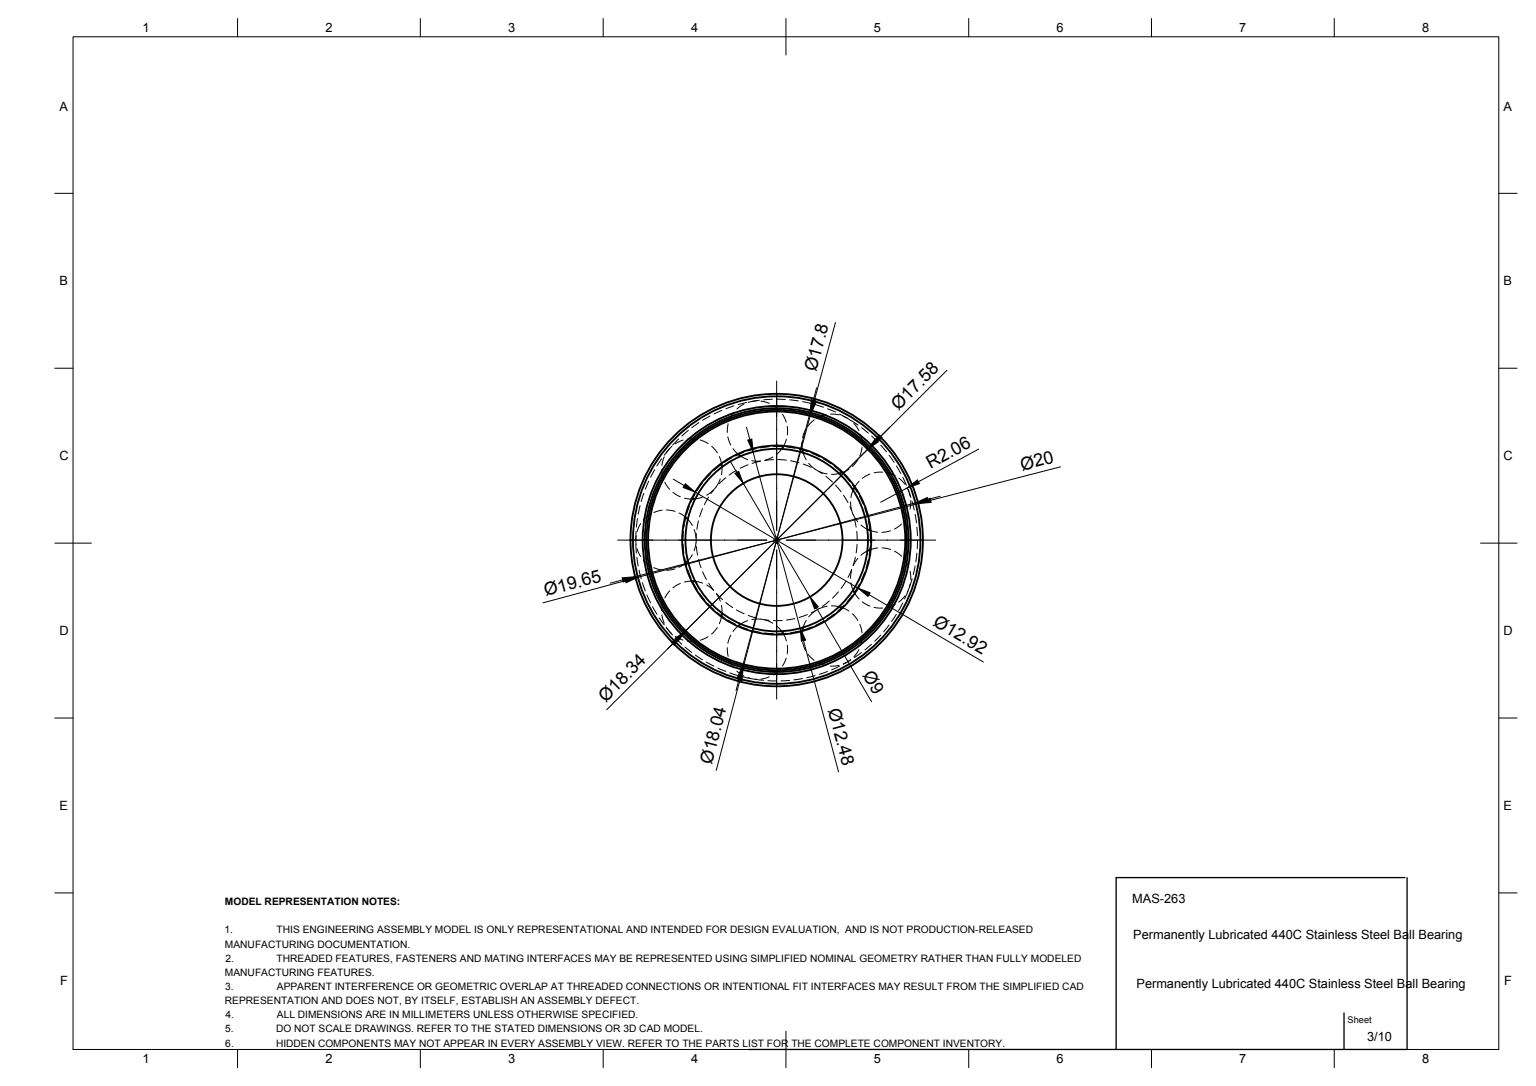
ISO-10303-21;
HEADER;
/* Generated by software containing ST-Developer
 * from STEP Tools, Inc. (www.steptools.com) 
 */

FILE_DESCRIPTION(
/* description */ (''),
/* implementation_level */ '2;1');

FILE_NAME(
/* name */ 'Permanently Lubricated 440C Stainless Steel Ball Bearing.step',
/* time_stamp */ '2026-10-12T15:47:30-07:00',
/* author */ (''),
/* organization */ (''),
/* preprocessor_version */ 'ST-DEVELOPER v20.2',
/* originating_system */ 'Autodesk Translation Framework v15.15.0.0',
/* authorisation */ '');

FILE_SCHEMA (('AUTOMOTIVE_DESIGN { 1 0 10303 214 3 1 1 }'));
ENDSEC;

DATA;
#10=MECHANICAL_DESIGN_GEOMETRIC_PRESENTATION_REPRESENTATION('',(#89,#90,#91,#92,#93,#94,#95,#96,#97,#98,#99,#100,#101,#102),#88483);
#55=SPHERICAL_SURFACE('',#14025,2.0625);
#56=SPHERICAL_SURFACE('',#14081,2.0625);
#57=SPHERICAL_SURFACE('',#14083,2.0625);
#58=SPHERICAL_SURFACE('',#14085,2.0625);
#59=SPHERICAL_SURFACE('',#14087,2.0625);
#60=SPHERICAL_SURFACE('',#14089,2.0625);
#61=SPHERICAL_SURFACE('',#14091,2.0625);
#62=SPHERICAL_SURFACE('',#14093,2.0625);
#63=SPHERICAL_SURFACE('',#14095,2.0625);
#71=SHAPE_REPRESENTATION_RELATIONSHIP('SRR','None',#88527,#80);
#80=ADVANCED_BREP_SHAPE_REPRESENTATION('',(#124,#125,#126,#127,#128,#129,
#130,#131,#132,#133,#134,#135,#136,#137),#88481);
#89=STYLED_ITEM('',(#88574),#124);
#90=STYLED_ITEM('',(#88574),#125);
#91=STYLED_ITEM('',(#88574),#126);
#92=STYLED_ITEM('',(#88574),#127);
#93=STYLED_ITEM('',(#88574),#128);
#94=STYLED_ITEM('',(#88574),#129);
#95=STYLED_ITEM('',(#88574),#130);
#96=STYLED_ITEM('',(#88574),#131);
#97=STYLED_ITEM('',(#88574),#132);
#98=STYLED_ITEM('',(#88574),#133);
#99=STYLED_ITEM('',(#88574),#134);
#100=STYLED_ITEM('',(#88574),#135);
#101=STYLED_ITEM('',(#88574),#136);
#102=STYLED_ITEM('',(#88574),#137);
#124=MANIFOLD_SOLID_BREP('Body1',#12999);
#125=MANIFOLD_SOLID_BREP('Body2',#13000);
#126=MANIFOLD_SOLID_BREP('Body3',#13001);
#127=MANIFOLD_SOLID_BREP('Body4',#13002);
#128=MANIFOLD_SOLID_BREP('Body5',#13003);
#129=MANIFOLD_SOLID_BREP('Body6',#13004);
#130=MANIFOLD_SOLID_BREP('Body7',#13005);
#131=MANIFOLD_SOLID_BREP('Body8',#13006);
#132=MANIFOLD_SOLID_BREP('Body9',#13007);
#133=MANIFOLD_SOLID_BREP('Body10',#13008);
#134=MANIFOLD_SOLID_BREP('Body11',#13009);
#135=MANIFOLD_SOLID_BREP('Body12',#13010);
#136=MANIFOLD_SOLID_BREP('Body13',#13011);
#137=MANIFOLD_SOLID_BREP('Body14',#13012);
#175=TOROIDAL_SURFACE('',#13994,7.57083333333333,2.0625);
#176=TOROIDAL_SURFACE('',#14007,5.00416666666667,0.260975870478375);
#177=TOROIDAL_SURFACE('',#14010,5.98069079618829,0.260975870478375);
#178=TOROIDAL_SURFACE('',#14017,5.98069079618829,0.260975870478375);
#179=TOROIDAL_SURFACE('',#14020,5.00416666666667,0.260975870478376);
#180=TOROIDAL_SURFACE('',#14030,6.50566666666666,0.0439999999999998);
#181=TOROIDAL_SURFACE('',#14047,6.50566666666666,0.0439999999999998);
#182=TOROIDAL_SURFACE('',#14075,7.57083333333333,2.0625);
#183=TOROIDAL_SURFACE('',#14100,6.32416666666667,0.0824999999999997);
#184=TOROIDAL_SURFACE('',#14105,6.42956528249449,0.0228986158278278);
#326=CONICAL_SURFACE('',#13998,4.5,0.26179938779915);
#327=CONICAL_SURFACE('',#14005,4.75208333333333,0.261799387799149);
#328=CONICAL_SURFACE('',#14033,8.9,0.523598775598299);
#329=CONICAL_SURFACE('',#14050,8.79,0.523598775598297);
#330=CONICAL_SURFACE('',#14054,9.01847925309041,0.349065850398861);
#331=CONICAL_SURFACE('',#14057,9.16847925309041,0.78539816339744);
#332=CONICAL_SURFACE('',#14059,10.,0.523598775598291);
#333=CONICAL_SURFACE('',#14065,9.82679491924311,0.52359877559829);
#334=CONICAL_SURFACE('',#14067,9.0184792530904,0.78539816339744);
#335=CONICAL_SURFACE('',#14070,8.9,0.349065850398861);
#336=CONICAL_SURFACE('',#14109,6.46166666666667,0.17453292519942);
#407=FACE_BOUND('',#2047,.T.);
#408=FACE_BOUND('',#2049,.T.);
#409=FACE_BOUND('',#2056,.T.);
#410=FACE_BOUND('',#2058,.T.);
#411=FACE_BOUND('',#2064,.T.);
#412=FACE_BOUND('',#2066,.T.);
#413=FACE_BOUND('',#2078,.T.);
#414=FACE_BOUND('',#2080,.T.);
#415=FACE_BOUND('',#2096,.T.);
#553=PLANE('',#14023);
#554=PLANE('',#14024);
#555=PLANE('',#14039);
#556=PLANE('',#14040);
#557=PLANE('',#14052);
#558=PLANE('',#14053);
#559=PLANE('',#14079);
#560=PLANE('',#14080);
#561=PLANE('',#14114);
#1310=FACE_OUTER_BOUND('',#2036,.T.);
#1311=FACE_OUTER_BOUND('',#2037,.T.);
#1312=FACE_OUTER_BOUND('',#2038,.T.);
#1313=FACE_OUTER_BOUND('',#2039,.T.);
#1314=FACE_OUTER_BOUND('',#2040,.T.);
#1315=FACE_OUTER_BOUND('',#2041,.T.);
#1316=FACE_OUTER_BOUND('',#2042,.T.);
#1317=FACE_OUTER_BOUND('',#2043,.T.);
#1318=FACE_OUTER_BOUND('',#2044,.T.);
#1319=FACE_OUTER_BOUND('',#2045,.T.);
#1320=FACE_OUTER_BOUND('',#2046,.T.);
#1321=FACE_OUTER_BOUND('',#2048,.T.);
#1322=FACE_OUTER_BOUND('',#2050,.T.);
#1323=FACE_OUTER_BOUND('',#2051,.T.);
#1324=FACE_OUTER_BOUND('',#2052,.T.);
#1325=FACE_OUTER_BOUND('',#2053,.T.);
#1326=FACE_OUTER_BOUND('',#2054,.T.);
#1327=FACE_OUTER_BOUND('',#2055,.T.);
#1328=FACE_OUTER_BOUND('',#2057,.T.);
#1329=FACE_OUTER_BOUND('',#2059,.T.);
#1330=FACE_OUTER_BOUND('',#2060,.T.);
#1331=FACE_OUTER_BOUND('',#2061,.T.);
#1332=FACE_OUTER_BOUND('',#2062,.T.);
#1333=FACE_OUTER_BOUND('',#2063,.T.);
#1334=FACE_OUTER_BOUND('',#2065,.T.);
#1335=FACE_OUTER_BOUND('',#2067,.T.);
#1336=FACE_OUTER_BOUND('',#2068,.T.);
#1337=FACE_OUTER_BOUND('',#2069,.T.);
#1338=FACE_OUTER_BOUND('',#2070,.T.);
#1339=FACE_OUTER_BOUND('',#2071,.T.);
#1340=FACE_OUTER_BOUND('',#2072,.T.);
#1341=FACE_OUTER_BOUND('',#2073,.T.);
#1342=FACE_OUTER_BOUND('',#2074,.T.);
#1343=FACE_OUTER_BOUND('',#2075,.T.);
#1344=FACE_OUTER_BOUND('',#2076,.T.);
#1345=FACE_OUTER_BOUND('',#2077,.T.);
#1346=FACE_OUTER_BOUND('',#2079,.T.);
#1347=FACE_OUTER_BOUND('',#2081,.T.);
#1348=FACE_OUTER_BOUND('',#2082,.T.);
#1349=FACE_OUTER_BOUND('',#2083,.T.);
#1350=FACE_OUTER_BOUND('',#2084,.T.);
#1351=FACE_OUTER_BOUND('',#2085,.T.);
#1352=FACE_OUTER_BOUND('',#2086,.T.);
#1353=FACE_OUTER_BOUND('',#2087,.T.);
#1354=FACE_OUTER_BOUND('',#2088,.T.);
#1355=FACE_OUTER_BOUND('',#2089,.T.);
#1356=FACE_OUTER_BOUND('',#2090,.T.);
#1357=FACE_OUTER_BOUND('',#2091,.T.);
#1358=FACE_OUTER_BOUND('',#2092,.T.);
#1359=FACE_OUTER_BOUND('',#2093,.T.);
#1360=FACE_OUTER_BOUND('',#2094,.T.);
#1361=FACE_OUTER_BOUND('',#2095,.T.);
#2036=EDGE_LOOP('',(#11488,#11489,#11490,#11491));
#2037=EDGE_LOOP('',(#11492,#11493,#11494,#11495,#11496,#11497));
#2038=EDGE_LOOP('',(#11498,#11499,#11500,#11501,#11502));
#2039=EDGE_LOOP('',(#11503,#11504,#11505,#11506));
#2040=EDGE_LOOP('',(#11507,#11508,#11509,#11510));
#2041=EDGE_LOOP('',(#11511,#11512,#11513,#11514));
#2042=EDGE_LOOP('',(#11515,#11516,#11517,#11518));
#2043=EDGE_LOOP('',(#11519,#11520,#11521,#11522));
#2044=EDGE_LOOP('',(#11523,#11524,#11525,#11526));
#2045=EDGE_LOOP('',(#11527,#11528,#11529,#11530,#11531));
#2046=EDGE_LOOP('',(#11532));
#2047=EDGE_LOOP('',(#11533));
#2048=EDGE_LOOP('',(#11534));
#2049=EDGE_LOOP('',(#11535));
#2050=EDGE_LOOP('',(#11536,#11537));
#2051=EDGE_LOOP('',(#11538,#11539,#11540,#11541));
#2052=EDGE_LOOP('',(#11542,#11543,#11544,#11545));
#2053=EDGE_LOOP('',(#11546,#11547,#11548,#11549,#11550));
#2054=EDGE_LOOP('',(#11551,#11552,#11553,#11554,#11555));
#2055=EDGE_LOOP('',(#11556));
#2056=EDGE_LOOP('',(#11557));
#2057=EDGE_LOOP('',(#11558));
#2058=EDGE_LOOP('',(#11559));
#2059=EDGE_LOOP('',(#11560,#11561,#11562,#11563));
#2060=EDGE_LOOP('',(#11564,#11565,#11566,#11567));
#2061=EDGE_LOOP('',(#11568,#11569,#11570,#11571));
#2062=EDGE_LOOP('',(#11572,#11573,#11574,#11575));
#2063=EDGE_LOOP('',(#11576));
#2064=EDGE_LOOP('',(#11577));
#2065=EDGE_LOOP('',(#11578));
#2066=EDGE_LOOP('',(#11579));
#2067=EDGE_LOOP('',(#11580,#11581,#11582,#11583));
#2068=EDGE_LOOP('',(#11584,#11585,#11586,#11587));
#2069=EDGE_LOOP('',(#11588,#11589,#11590,#11591,#11592));
#2070=EDGE_LOOP('',(#11593,#11594,#11595,#11596,#11597));
#2071=EDGE_LOOP('',(#11598,#11599,#11600,#11601));
#2072=EDGE_LOOP('',(#11602,#11603,#11604,#11605));
#2073=EDGE_LOOP('',(#11606,#11607,#11608,#11609,#11610));
#2074=EDGE_LOOP('',(#11611,#11612,#11613,#11614,#11615));
#2075=EDGE_LOOP('',(#11616,#11617,#11618,#11619));
#2076=EDGE_LOOP('',(#11620,#11621,#11622,#11623));
#2077=EDGE_LOOP('',(#11624));
#2078=EDGE_LOOP('',(#11625));
#2079=EDGE_LOOP('',(#11626));
#2080=EDGE_LOOP('',(#11627));
#2081=EDGE_LOOP('',(#11628,#11629));
#2082=EDGE_LOOP('',(#11630,#11631));
#2083=EDGE_LOOP('',(#11632,#11633));
#2084=EDGE_LOOP('',(#11634,#11635));
#2085=EDGE_LOOP('',(#11636,#11637));
#2086=EDGE_LOOP('',(#11638,#11639));
#2087=EDGE_LOOP('',(#11640,#11641));
#2088=EDGE_LOOP('',(#11642,#11643));
#2089=EDGE_LOOP('',(#11644,#11645,#11646,#11647));
#2090=EDGE_LOOP('',(#11648,#11649,#11650,#11651));
#2091=EDGE_LOOP('',(#11652,#11653,#11654,#11655));
#2092=EDGE_LOOP('',(#11656,#11657,#11658,#11659,#11660));
#2093=EDGE_LOOP('',(#11661,#11662,#11663,#11664,#11665,#11666));
#2094=EDGE_LOOP('',(#11667,#11668,#11669,#11670,#11671));
#2095=EDGE_LOOP('',(#11672));
#2096=EDGE_LOOP('',(#11673));
#2699=CIRCLE('',#13995,6.24166666666667);
#2700=CIRCLE('',#13996,2.0625);
#2701=CIRCLE('',#13997,6.24166666666667);
#2702=CIRCLE('',#13999,4.5);
#2703=CIRCLE('',#14000,4.75208333333333);
#2704=CIRCLE('',#14001,4.75208333333333);
#2705=CIRCLE('',#14002,4.5);
#2706=CIRCLE('',#14004,4.5);
#2707=CIRCLE('',#14006,4.75208333333333);
#2708=CIRCLE('',#14008,0.260975870478375);
#2709=CIRCLE('',#14009,5.00416666666667);
#2710=CIRCLE('',#14011,5.98069079618829);
#2711=CIRCLE('',#14012,0.260975870478375);
#2712=CIRCLE('',#14013,6.24166666666667);
#2713=CIRCLE('',#14016,6.24166666666667);
#2714=CIRCLE('',#14018,0.260975870478375);
#2715=CIRCLE('',#14019,5.98069079618829);
#2716=CIRCLE('',#14021,5.00416666666667);
#2717=CIRCLE('',#14022,0.260975870478376);
#2718=CIRCLE('',#14026,2.0625);
#2719=CIRCLE('',#14028,6.46166666666667);
#2720=CIRCLE('',#14029,6.46166666666667);
#2721=CIRCLE('',#14031,0.0439999999999998);
#2722=CIRCLE('',#14032,6.50566666666666);
#2723=CIRCLE('',#14034,8.9);
#2724=CIRCLE('',#14035,8.79);
#2725=CIRCLE('',#14036,8.9);
#2726=CIRCLE('',#14038,8.9);
#2727=CIRCLE('',#14042,8.9);
#2728=CIRCLE('',#14043,8.9);
#2729=CIRCLE('',#14045,6.46166666666667);
#2730=CIRCLE('',#14046,6.46166666666667);
#2731=CIRCLE('',#14048,6.50566666666666);
#2732=CIRCLE('',#14049,0.0439999999999998);
#2733=CIRCLE('',#14051,8.79);
#2734=CIRCLE('',#14055,8.9);
#2735=CIRCLE('',#14056,9.01847925309041);
#2736=CIRCLE('',#14058,9.16847925309041);
#2737=CIRCLE('',#14060,10.);
#2738=CIRCLE('',#14061,9.82679491924311);
#2739=CIRCLE('',#14062,10.);
#2740=CIRCLE('',#14064,10.);
#2741=CIRCLE('',#14066,9.82679491924311);
#2742=CIRCLE('',#14068,9.0184792530904);
#2743=CIRCLE('',#14069,9.1684792530904);
#2744=CIRCLE('',#14071,8.9);
#2745=CIRCLE('',#14072,8.9);
#2746=CIRCLE('',#14074,8.9);
#2747=CIRCLE('',#14076,2.0625);
#2748=CIRCLE('',#14077,8.9);
#2749=CIRCLE('',#14082,2.0625);
#2750=CIRCLE('',#14084,2.0625);
#2751=CIRCLE('',#14086,2.0625);
#2752=CIRCLE('',#14088,2.0625);
#2753=CIRCLE('',#14090,2.0625);
#2754=CIRCLE('',#14092,2.0625);
#2755=CIRCLE('',#14094,2.0625);
#2756=CIRCLE('',#14096,2.0625);
#2757=CIRCLE('',#14098,6.24166666666667);
#2758=CIRCLE('',#14099,6.24166666666667);
#2759=CIRCLE('',#14101,0.0824999999999997);
#2760=CIRCLE('',#14102,6.40666666666666);
#2761=CIRCLE('',#14104,6.40666666666667);
#2762=CIRCLE('',#14106,0.0228986158278278);
#2763=CIRCLE('',#14107,6.45211601689499);
#2764=CIRCLE('',#14108,6.45211601689499);
#2765=CIRCLE('',#14110,6.46166666666667);
#2766=CIRCLE('',#14111,6.46166666666667);
#2767=CIRCLE('',#14113,6.46166666666667);
#4094=LINE('',#87514,#4564);
#4095=LINE('',#87521,#4565);
#4096=LINE('',#87525,#4566);
#4097=LINE('',#87538,#4567);
#4098=LINE('',#87541,#4568);
#4099=LINE('',#87561,#4569);
#4100=LINE('',#87572,#4570);
#4101=LINE('',#87577,#4571);
#4102=LINE('',#87585,#4572);
#4103=LINE('',#87591,#4573);
#4104=LINE('',#87599,#4574);
#4105=LINE('',#87607,#4575);
#4106=LINE('',#87611,#4576);
#4107=LINE('',#87618,#4577);
#4108=LINE('',#87623,#4578);
#4109=LINE('',#87627,#4579);
#4110=LINE('',#87633,#4580);
#4111=LINE('',#87639,#4581);
#4112=LINE('',#87643,#4582);
#4113=LINE('',#87650,#4583);
#4114=LINE('',#87689,#4584);
#4115=LINE('',#87697,#4585);
#4116=LINE('',#87709,#4586);
#4117=LINE('',#87713,#4587);
#4564=VECTOR('',#16544,4.5);
#4565=VECTOR('',#16553,4.5);
#4566=VECTOR('',#16558,4.75208333333333);
#4567=VECTOR('',#16577,6.24166666666667);
#4568=VECTOR('',#16580,6.24166666666667);
#4569=VECTOR('',#16607,6.46166666666667);
#4570=VECTOR('',#16620,8.9);
#4571=VECTOR('',#16627,8.9);
#4572=VECTOR('',#16638,8.9);
#4573=VECTOR('',#16645,6.46166666666667);
#4574=VECTOR('',#16656,8.79);
#4575=VECTOR('',#16667,9.01847925309041);
#4576=VECTOR('',#16672,9.16847925309041);
#4577=VECTOR('',#16679,10.);
#4578=VECTOR('',#16686,10.);
#4579=VECTOR('',#16691,9.82679491924311);
#4580=VECTOR('',#16698,9.0184792530904);
#4581=VECTOR('',#16705,8.9);
#4582=VECTOR('',#16710,8.9);
#4583=VECTOR('',#16721,8.9);
#4584=VECTOR('',#16762,6.24166666666667);
#4585=VECTOR('',#16773,6.40666666666667);
#4586=VECTOR('',#16788,6.46166666666667);
#4587=VECTOR('',#16793,6.46166666666667);
#5833=VERTEX_POINT('',#87504);
#5834=VERTEX_POINT('',#87506);
#5835=VERTEX_POINT('',#87510);
#5836=VERTEX_POINT('',#87511);
#5837=VERTEX_POINT('',#87513);
#5838=VERTEX_POINT('',#87515);
#5839=VERTEX_POINT('',#87520);
#5840=VERTEX_POINT('',#87524);
#5841=VERTEX_POINT('',#87528);
#5842=VERTEX_POINT('',#87532);
#5843=VERTEX_POINT('',#87534);
#5844=VERTEX_POINT('',#87540);
#5845=VERTEX_POINT('',#87544);
#5846=VERTEX_POINT('',#87548);
#5847=VERTEX_POINT('',#87554);
#5848=VERTEX_POINT('',#87555);
#5849=VERTEX_POINT('',#87558);
#5850=VERTEX_POINT('',#87560);
#5851=VERTEX_POINT('',#87564);
#5852=VERTEX_POINT('',#87568);
#5853=VERTEX_POINT('',#87569);
#5854=VERTEX_POINT('',#87571);
#5855=VERTEX_POINT('',#87576);
#5856=VERTEX_POINT('',#87582);
#5857=VERTEX_POINT('',#87584);
#5858=VERTEX_POINT('',#87588);
#5859=VERTEX_POINT('',#87590);
#5860=VERTEX_POINT('',#87594);
#5861=VERTEX_POINT('',#87598);
#5862=VERTEX_POINT('',#87604);
#5863=VERTEX_POINT('',#87606);
#5864=VERTEX_POINT('',#87610);
#5865=VERTEX_POINT('',#87614);
#5866=VERTEX_POINT('',#87615);
#5867=VERTEX_POINT('',#87617);
#5868=VERTEX_POINT('',#87622);
#5869=VERTEX_POINT('',#87626);
#5870=VERTEX_POINT('',#87630);
#5871=VERTEX_POINT('',#87632);
#5872=VERTEX_POINT('',#87636);
#5873=VERTEX_POINT('',#87637);
#5874=VERTEX_POINT('',#87642);
#5875=VERTEX_POINT('',#87646);
#5876=VERTEX_POINT('',#87654);
#5877=VERTEX_POINT('',#87655);
#5878=VERTEX_POINT('',#87658);
#5879=VERTEX_POINT('',#87659);
#5880=VERTEX_POINT('',#87662);
#5881=VERTEX_POINT('',#87663);
#5882=VERTEX_POINT('',#87666);
#5883=VERTEX_POINT('',#87667);
#5884=VERTEX_POINT('',#87670);
#5885=VERTEX_POINT('',#87671);
#5886=VERTEX_POINT('',#87674);
#5887=VERTEX_POINT('',#87675);
#5888=VERTEX_POINT('',#87678);
#5889=VERTEX_POINT('',#87679);
#5890=VERTEX_POINT('',#87682);
#5891=VERTEX_POINT('',#87683);
#5892=VERTEX_POINT('',#87686);
#5893=VERTEX_POINT('',#87688);
#5894=VERTEX_POINT('',#87692);
#5895=VERTEX_POINT('',#87696);
#5896=VERTEX_POINT('',#87700);
#5897=VERTEX_POINT('',#87702);
#5898=VERTEX_POINT('',#87706);
#5899=VERTEX_POINT('',#87707);
#5900=VERTEX_POINT('',#87712);
#7756=EDGE_CURVE('',#5833,#5833,#2699,.T.);
#7757=EDGE_CURVE('',#5833,#5834,#2700,.T.);
#7758=EDGE_CURVE('',#5834,#5834,#2701,.T.);
#7759=EDGE_CURVE('',#5835,#5836,#2702,.T.);
#7760=EDGE_CURVE('',#5836,#5837,#4094,.T.);
#7761=EDGE_CURVE('',#5838,#5837,#2703,.T.);
#7762=EDGE_CURVE('',#5837,#5838,#2704,.T.);
#7763=EDGE_CURVE('',#5836,#5835,#2705,.T.);
#7764=EDGE_CURVE('',#5835,#5839,#4095,.T.);
#7765=EDGE_CURVE('',#5839,#5839,#2706,.T.);
#7766=EDGE_CURVE('',#5839,#5840,#4096,.T.);
#7767=EDGE_CURVE('',#5840,#5840,#2707,.T.);
#7768=EDGE_CURVE('',#5840,#5841,#2708,.T.);
#7769=EDGE_CURVE('',#5841,#5841,#2709,.T.);
#7770=EDGE_CURVE('',#5842,#5842,#2710,.T.);
#7771=EDGE_CURVE('',#5842,#5843,#2711,.T.);
#7772=EDGE_CURVE('',#5843,#5843,#2712,.T.);
#7773=EDGE_CURVE('',#5843,#5833,#4097,.T.);
#7774=EDGE_CURVE('',#5834,#5844,#4098,.T.);
#7775=EDGE_CURVE('',#5844,#5844,#2713,.T.);
#7776=EDGE_CURVE('',#5844,#5845,#2714,.T.);
#7777=EDGE_CURVE('',#5845,#5845,#2715,.T.);
#7778=EDGE_CURVE('',#5846,#5846,#2716,.T.);
#7779=EDGE_CURVE('',#5846,#5838,#2717,.T.);
#7780=EDGE_CURVE('',#5847,#5848,#2718,.T.);
#7781=EDGE_CURVE('',#5849,#5849,#2719,.T.);
#7782=EDGE_CURVE('',#5849,#5850,#4099,.T.);
#7783=EDGE_CURVE('',#5850,#5850,#2720,.T.);
#7784=EDGE_CURVE('',#5850,#5851,#2721,.T.);
#7785=EDGE_CURVE('',#5851,#5851,#2722,.T.);
#7786=EDGE_CURVE('',#5852,#5853,#2723,.T.);
#7787=EDGE_CURVE('',#5853,#5854,#4100,.T.);
#7788=EDGE_CURVE('',#5854,#5854,#2724,.T.);
#7789=EDGE_CURVE('',#5853,#5852,#2725,.T.);
#7790=EDGE_CURVE('',#5852,#5855,#4101,.T.);
#7791=EDGE_CURVE('',#5855,#5855,#2726,.T.);
#7792=EDGE_CURVE('',#5856,#5856,#2727,.T.);
#7793=EDGE_CURVE('',#5856,#5857,#4102,.T.);
#7794=EDGE_CURVE('',#5857,#5857,#2728,.T.);
#7795=EDGE_CURVE('',#5858,#5858,#2729,.T.);
#7796=EDGE_CURVE('',#5858,#5859,#4103,.T.);
#7797=EDGE_CURVE('',#5859,#5859,#2730,.T.);
#7798=EDGE_CURVE('',#5860,#5860,#2731,.T.);
#7799=EDGE_CURVE('',#5860,#5858,#2732,.T.);
#7800=EDGE_CURVE('',#5857,#5861,#4104,.T.);
#7801=EDGE_CURVE('',#5861,#5861,#2733,.T.);
#7802=EDGE_CURVE('',#5862,#5862,#2734,.T.);
#7803=EDGE_CURVE('',#5862,#5863,#4105,.T.);
#7804=EDGE_CURVE('',#5863,#5863,#2735,.T.);
#7805=EDGE_CURVE('',#5863,#5864,#4106,.T.);
#7806=EDGE_CURVE('',#5864,#5864,#2736,.T.);
#7807=EDGE_CURVE('',#5865,#5866,#2737,.T.);
#7808=EDGE_CURVE('',#5866,#5867,#4107,.T.);
#7809=EDGE_CURVE('',#5867,#5867,#2738,.T.);
#7810=EDGE_CURVE('',#5866,#5865,#2739,.T.);
#7811=EDGE_CURVE('',#5865,#5868,#4108,.T.);
#7812=EDGE_CURVE('',#5868,#5868,#2740,.T.);
#7813=EDGE_CURVE('',#5868,#5869,#4109,.T.);
#7814=EDGE_CURVE('',#5869,#5869,#2741,.T.);
#7815=EDGE_CURVE('',#5870,#5870,#2742,.T.);
#7816=EDGE_CURVE('',#5870,#5871,#4110,.T.);
#7817=EDGE_CURVE('',#5871,#5871,#2743,.T.);
#7818=EDGE_CURVE('',#5872,#5873,#2744,.T.);
#7819=EDGE_CURVE('',#5873,#5870,#4111,.T.);
#7820=EDGE_CURVE('',#5873,#5872,#2745,.T.);
#7821=EDGE_CURVE('',#5872,#5874,#4112,.T.);
#7822=EDGE_CURVE('',#5874,#5874,#2746,.T.);
#7823=EDGE_CURVE('',#5874,#5875,#2747,.T.);
#7824=EDGE_CURVE('',#5875,#5875,#2748,.T.);
#7825=EDGE_CURVE('',#5875,#5862,#4113,.T.);
#7826=EDGE_CURVE('',#5876,#5877,#2749,.T.);
#7827=EDGE_CURVE('',#5878,#5879,#2750,.T.);
#7828=EDGE_CURVE('',#5880,#5881,#2751,.T.);
#7829=EDGE_CURVE('',#5882,#5883,#2752,.T.);
#7830=EDGE_CURVE('',#5884,#5885,#2753,.T.);
#7831=EDGE_CURVE('',#5886,#5887,#2754,.T.);
#7832=EDGE_CURVE('',#5888,#5889,#2755,.T.);
#7833=EDGE_CURVE('',#5890,#5891,#2756,.T.);
#7834=EDGE_CURVE('',#5892,#5892,#2757,.T.);
#7835=EDGE_CURVE('',#5892,#5893,#4114,.T.);
#7836=EDGE_CURVE('',#5893,#5893,#2758,.T.);
#7837=EDGE_CURVE('',#5893,#5894,#2759,.T.);
#7838=EDGE_CURVE('',#5894,#5894,#2760,.T.);
#7839=EDGE_CURVE('',#5894,#5895,#4115,.T.);
#7840=EDGE_CURVE('',#5895,#5895,#2761,.T.);
#7841=EDGE_CURVE('',#5895,#5896,#2762,.T.);
#7842=EDGE_CURVE('',#5896,#5897,#2763,.T.);
#7843=EDGE_CURVE('',#5897,#5896,#2764,.T.);
#7844=EDGE_CURVE('',#5898,#5899,#2765,.T.);
#7845=EDGE_CURVE('',#5899,#5897,#4116,.T.);
#7846=EDGE_CURVE('',#5899,#5898,#2766,.T.);
#7847=EDGE_CURVE('',#5898,#5900,#4117,.T.);
#7848=EDGE_CURVE('',#5900,#5900,#2767,.T.);
#11488=ORIENTED_EDGE('',*,*,#7756,.F.);
#11489=ORIENTED_EDGE('',*,*,#7757,.T.);
#11490=ORIENTED_EDGE('',*,*,#7758,.T.);
#11491=ORIENTED_EDGE('',*,*,#7757,.F.);
#11492=ORIENTED_EDGE('',*,*,#7759,.T.);
#11493=ORIENTED_EDGE('',*,*,#7760,.T.);
#11494=ORIENTED_EDGE('',*,*,#7761,.F.);
#11495=ORIENTED_EDGE('',*,*,#7762,.F.);
#11496=ORIENTED_EDGE('',*,*,#7760,.F.);
#11497=ORIENTED_EDGE('',*,*,#7763,.T.);
#11498=ORIENTED_EDGE('',*,*,#7759,.F.);
#11499=ORIENTED_EDGE('',*,*,#7764,.T.);
#11500=ORIENTED_EDGE('',*,*,#7765,.T.);
#11501=ORIENTED_EDGE('',*,*,#7764,.F.);
#11502=ORIENTED_EDGE('',*,*,#7763,.F.);
#11503=ORIENTED_EDGE('',*,*,#7765,.F.);
#11504=ORIENTED_EDGE('',*,*,#7766,.T.);
#11505=ORIENTED_EDGE('',*,*,#7767,.T.);
#11506=ORIENTED_EDGE('',*,*,#7766,.F.);
#11507=ORIENTED_EDGE('',*,*,#7767,.F.);
#11508=ORIENTED_EDGE('',*,*,#7768,.T.);
#11509=ORIENTED_EDGE('',*,*,#7769,.T.);
#11510=ORIENTED_EDGE('',*,*,#7768,.F.);
#11511=ORIENTED_EDGE('',*,*,#7770,.F.);
#11512=ORIENTED_EDGE('',*,*,#7771,.T.);
#11513=ORIENTED_EDGE('',*,*,#7772,.T.);
#11514=ORIENTED_EDGE('',*,*,#7771,.F.);
#11515=ORIENTED_EDGE('',*,*,#7772,.F.);
#11516=ORIENTED_EDGE('',*,*,#7773,.T.);
#11517=ORIENTED_EDGE('',*,*,#7756,.T.);
#11518=ORIENTED_EDGE('',*,*,#7773,.F.);
#11519=ORIENTED_EDGE('',*,*,#7758,.F.);
#11520=ORIENTED_EDGE('',*,*,#7774,.T.);
#11521=ORIENTED_EDGE('',*,*,#7775,.T.);
#11522=ORIENTED_EDGE('',*,*,#7774,.F.);
#11523=ORIENTED_EDGE('',*,*,#7775,.F.);
#11524=ORIENTED_EDGE('',*,*,#7776,.T.);
#11525=ORIENTED_EDGE('',*,*,#7777,.T.);
#11526=ORIENTED_EDGE('',*,*,#7776,.F.);
#11527=ORIENTED_EDGE('',*,*,#7778,.F.);
#11528=ORIENTED_EDGE('',*,*,#7779,.T.);
#11529=ORIENTED_EDGE('',*,*,#7761,.T.);
#11530=ORIENTED_EDGE('',*,*,#7762,.T.);
#11531=ORIENTED_EDGE('',*,*,#7779,.F.);
#11532=ORIENTED_EDGE('',*,*,#7777,.F.);
#11533=ORIENTED_EDGE('',*,*,#7778,.T.);
#11534=ORIENTED_EDGE('',*,*,#7770,.T.);
#11535=ORIENTED_EDGE('',*,*,#7769,.F.);
#11536=ORIENTED_EDGE('',*,*,#7780,.T.);
#11537=ORIENTED_EDGE('',*,*,#7780,.F.);
#11538=ORIENTED_EDGE('',*,*,#7781,.F.);
#11539=ORIENTED_EDGE('',*,*,#7782,.T.);
#11540=ORIENTED_EDGE('',*,*,#7783,.T.);
#11541=ORIENTED_EDGE('',*,*,#7782,.F.);
#11542=ORIENTED_EDGE('',*,*,#7783,.F.);
#11543=ORIENTED_EDGE('',*,*,#7784,.T.);
#11544=ORIENTED_EDGE('',*,*,#7785,.T.);
#11545=ORIENTED_EDGE('',*,*,#7784,.F.);
#11546=ORIENTED_EDGE('',*,*,#7786,.T.);
#11547=ORIENTED_EDGE('',*,*,#7787,.T.);
#11548=ORIENTED_EDGE('',*,*,#7788,.F.);
#11549=ORIENTED_EDGE('',*,*,#7787,.F.);
#11550=ORIENTED_EDGE('',*,*,#7789,.T.);
#11551=ORIENTED_EDGE('',*,*,#7786,.F.);
#11552=ORIENTED_EDGE('',*,*,#7790,.T.);
#11553=ORIENTED_EDGE('',*,*,#7791,.T.);
#11554=ORIENTED_EDGE('',*,*,#7790,.F.);
#11555=ORIENTED_EDGE('',*,*,#7789,.F.);
#11556=ORIENTED_EDGE('',*,*,#7791,.F.);
#11557=ORIENTED_EDGE('',*,*,#7781,.T.);
#11558=ORIENTED_EDGE('',*,*,#7788,.T.);
#11559=ORIENTED_EDGE('',*,*,#7785,.F.);
#11560=ORIENTED_EDGE('',*,*,#7792,.F.);
#11561=ORIENTED_EDGE('',*,*,#7793,.T.);
#11562=ORIENTED_EDGE('',*,*,#7794,.T.);
#11563=ORIENTED_EDGE('',*,*,#7793,.F.);
#11564=ORIENTED_EDGE('',*,*,#7795,.F.);
#11565=ORIENTED_EDGE('',*,*,#7796,.T.);
#11566=ORIENTED_EDGE('',*,*,#7797,.T.);
#11567=ORIENTED_EDGE('',*,*,#7796,.F.);
#11568=ORIENTED_EDGE('',*,*,#7798,.F.);
#11569=ORIENTED_EDGE('',*,*,#7799,.T.);
#11570=ORIENTED_EDGE('',*,*,#7795,.T.);
#11571=ORIENTED_EDGE('',*,*,#7799,.F.);
#11572=ORIENTED_EDGE('',*,*,#7794,.F.);
#11573=ORIENTED_EDGE('',*,*,#7800,.T.);
#11574=ORIENTED_EDGE('',*,*,#7801,.T.);
#11575=ORIENTED_EDGE('',*,*,#7800,.F.);
#11576=ORIENTED_EDGE('',*,*,#7801,.F.);
#11577=ORIENTED_EDGE('',*,*,#7798,.T.);
#11578=ORIENTED_EDGE('',*,*,#7792,.T.);
#11579=ORIENTED_EDGE('',*,*,#7797,.F.);
#11580=ORIENTED_EDGE('',*,*,#7802,.F.);
#11581=ORIENTED_EDGE('',*,*,#7803,.T.);
#11582=ORIENTED_EDGE('',*,*,#7804,.T.);
#11583=ORIENTED_EDGE('',*,*,#7803,.F.);
#11584=ORIENTED_EDGE('',*,*,#7804,.F.);
#11585=ORIENTED_EDGE('',*,*,#7805,.T.);
#11586=ORIENTED_EDGE('',*,*,#7806,.T.);
#11587=ORIENTED_EDGE('',*,*,#7805,.F.);
#11588=ORIENTED_EDGE('',*,*,#7807,.T.);
#11589=ORIENTED_EDGE('',*,*,#7808,.T.);
#11590=ORIENTED_EDGE('',*,*,#7809,.F.);
#11591=ORIENTED_EDGE('',*,*,#7808,.F.);
#11592=ORIENTED_EDGE('',*,*,#7810,.T.);
#11593=ORIENTED_EDGE('',*,*,#7807,.F.);
#11594=ORIENTED_EDGE('',*,*,#7811,.T.);
#11595=ORIENTED_EDGE('',*,*,#7812,.T.);
#11596=ORIENTED_EDGE('',*,*,#7811,.F.);
#11597=ORIENTED_EDGE('',*,*,#7810,.F.);
#11598=ORIENTED_EDGE('',*,*,#7812,.F.);
#11599=ORIENTED_EDGE('',*,*,#7813,.T.);
#11600=ORIENTED_EDGE('',*,*,#7814,.T.);
#11601=ORIENTED_EDGE('',*,*,#7813,.F.);
#11602=ORIENTED_EDGE('',*,*,#7815,.T.);
#11603=ORIENTED_EDGE('',*,*,#7816,.T.);
#11604=ORIENTED_EDGE('',*,*,#7817,.F.);
#11605=ORIENTED_EDGE('',*,*,#7816,.F.);
#11606=ORIENTED_EDGE('',*,*,#7818,.T.);
#11607=ORIENTED_EDGE('',*,*,#7819,.T.);
#11608=ORIENTED_EDGE('',*,*,#7815,.F.);
#11609=ORIENTED_EDGE('',*,*,#7819,.F.);
#11610=ORIENTED_EDGE('',*,*,#7820,.T.);
#11611=ORIENTED_EDGE('',*,*,#7818,.F.);
#11612=ORIENTED_EDGE('',*,*,#7821,.T.);
#11613=ORIENTED_EDGE('',*,*,#7822,.T.);
#11614=ORIENTED_EDGE('',*,*,#7821,.F.);
#11615=ORIENTED_EDGE('',*,*,#7820,.F.);
#11616=ORIENTED_EDGE('',*,*,#7822,.F.);
#11617=ORIENTED_EDGE('',*,*,#7823,.T.);
#11618=ORIENTED_EDGE('',*,*,#7824,.T.);
#11619=ORIENTED_EDGE('',*,*,#7823,.F.);
#11620=ORIENTED_EDGE('',*,*,#7824,.F.);
#11621=ORIENTED_EDGE('',*,*,#7825,.T.);
#11622=ORIENTED_EDGE('',*,*,#7802,.T.);
#11623=ORIENTED_EDGE('',*,*,#7825,.F.);
#11624=ORIENTED_EDGE('',*,*,#7814,.F.);
#11625=ORIENTED_EDGE('',*,*,#7817,.T.);
#11626=ORIENTED_EDGE('',*,*,#7809,.T.);
#11627=ORIENTED_EDGE('',*,*,#7806,.F.);
#11628=ORIENTED_EDGE('',*,*,#7826,.T.);
#11629=ORIENTED_EDGE('',*,*,#7826,.F.);
#11630=ORIENTED_EDGE('',*,*,#7827,.T.);
#11631=ORIENTED_EDGE('',*,*,#7827,.F.);
#11632=ORIENTED_EDGE('',*,*,#7828,.T.);
#11633=ORIENTED_EDGE('',*,*,#7828,.F.);
#11634=ORIENTED_EDGE('',*,*,#7829,.T.);
#11635=ORIENTED_EDGE('',*,*,#7829,.F.);
#11636=ORIENTED_EDGE('',*,*,#7830,.T.);
#11637=ORIENTED_EDGE('',*,*,#7830,.F.);
#11638=ORIENTED_EDGE('',*,*,#7831,.T.);
#11639=ORIENTED_EDGE('',*,*,#7831,.F.);
#11640=ORIENTED_EDGE('',*,*,#7832,.T.);
#11641=ORIENTED_EDGE('',*,*,#7832,.F.);
#11642=ORIENTED_EDGE('',*,*,#7833,.T.);
#11643=ORIENTED_EDGE('',*,*,#7833,.F.);
#11644=ORIENTED_EDGE('',*,*,#7834,.F.);
#11645=ORIENTED_EDGE('',*,*,#7835,.T.);
#11646=ORIENTED_EDGE('',*,*,#7836,.T.);
#11647=ORIENTED_EDGE('',*,*,#7835,.F.);
#11648=ORIENTED_EDGE('',*,*,#7836,.F.);
#11649=ORIENTED_EDGE('',*,*,#7837,.T.);
#11650=ORIENTED_EDGE('',*,*,#7838,.T.);
#11651=ORIENTED_EDGE('',*,*,#7837,.F.);
#11652=ORIENTED_EDGE('',*,*,#7838,.F.);
#11653=ORIENTED_EDGE('',*,*,#7839,.T.);
#11654=ORIENTED_EDGE('',*,*,#7840,.T.);
#11655=ORIENTED_EDGE('',*,*,#7839,.F.);
#11656=ORIENTED_EDGE('',*,*,#7840,.F.);
#11657=ORIENTED_EDGE('',*,*,#7841,.T.);
#11658=ORIENTED_EDGE('',*,*,#7842,.T.);
#11659=ORIENTED_EDGE('',*,*,#7843,.T.);
#11660=ORIENTED_EDGE('',*,*,#7841,.F.);
#11661=ORIENTED_EDGE('',*,*,#7844,.T.);
#11662=ORIENTED_EDGE('',*,*,#7845,.T.);
#11663=ORIENTED_EDGE('',*,*,#7842,.F.);
#11664=ORIENTED_EDGE('',*,*,#7843,.F.);
#11665=ORIENTED_EDGE('',*,*,#7845,.F.);
#11666=ORIENTED_EDGE('',*,*,#7846,.T.);
#11667=ORIENTED_EDGE('',*,*,#7844,.F.);
#11668=ORIENTED_EDGE('',*,*,#7847,.T.);
#11669=ORIENTED_EDGE('',*,*,#7848,.T.);
#11670=ORIENTED_EDGE('',*,*,#7847,.F.);
#11671=ORIENTED_EDGE('',*,*,#7846,.F.);
#11672=ORIENTED_EDGE('',*,*,#7848,.F.);
#11673=ORIENTED_EDGE('',*,*,#7834,.T.);
#12276=CYLINDRICAL_SURFACE('',#14003,4.5);
#12277=CYLINDRICAL_SURFACE('',#14014,6.24166666666667);
#12278=CYLINDRICAL_SURFACE('',#14015,6.24166666666667);
#12279=CYLINDRICAL_SURFACE('',#14027,6.46166666666667);
#12280=CYLINDRICAL_SURFACE('',#14037,8.9);
#12281=CYLINDRICAL_SURFACE('',#14041,8.9);
#12282=CYLINDRICAL_SURFACE('',#14044,6.46166666666667);
#12283=CYLINDRICAL_SURFACE('',#14063,10.);
#12284=CYLINDRICAL_SURFACE('',#14073,8.9);
#12285=CYLINDRICAL_SURFACE('',#14078,8.9);
#12286=CYLINDRICAL_SURFACE('',#14097,6.24166666666667);
#12287=CYLINDRICAL_SURFACE('',#14103,6.40666666666667);
#12288=CYLINDRICAL_SURFACE('',#14112,6.46166666666667);
#12840=ADVANCED_FACE('',(#1310),#175,.F.);
#12841=ADVANCED_FACE('',(#1311),#326,.F.);
#12842=ADVANCED_FACE('',(#1312),#12276,.F.);
#12843=ADVANCED_FACE('',(#1313),#327,.F.);
#12844=ADVANCED_FACE('',(#1314),#176,.T.);
#12845=ADVANCED_FACE('',(#1315),#177,.T.);
#12846=ADVANCED_FACE('',(#1316),#12277,.T.);
#12847=ADVANCED_FACE('',(#1317),#12278,.T.);
#12848=ADVANCED_FACE('',(#1318),#178,.T.);
#12849=ADVANCED_FACE('',(#1319),#179,.T.);
#12850=ADVANCED_FACE('',(#1320,#407),#553,.F.);
#12851=ADVANCED_FACE('',(#1321,#408),#554,.F.);
#12852=ADVANCED_FACE('',(#1322),#55,.T.);
#12853=ADVANCED_FACE('',(#1323),#12279,.F.);
#12854=ADVANCED_FACE('',(#1324),#180,.T.);
#12855=ADVANCED_FACE('',(#1325),#328,.T.);
#12856=ADVANCED_FACE('',(#1326),#12280,.T.);
#12857=ADVANCED_FACE('',(#1327,#409),#555,.F.);
#12858=ADVANCED_FACE('',(#1328,#410),#556,.F.);
#12859=ADVANCED_FACE('',(#1329),#12281,.T.);
#12860=ADVANCED_FACE('',(#1330),#12282,.F.);
#12861=ADVANCED_FACE('',(#1331),#181,.T.);
#12862=ADVANCED_FACE('',(#1332),#329,.T.);
#12863=ADVANCED_FACE('',(#1333,#411),#557,.F.);
#12864=ADVANCED_FACE('',(#1334,#412),#558,.F.);
#12865=ADVANCED_FACE('',(#1335),#330,.F.);
#12866=ADVANCED_FACE('',(#1336),#331,.F.);
#12867=ADVANCED_FACE('',(#1337),#332,.T.);
#12868=ADVANCED_FACE('',(#1338),#12283,.T.);
#12869=ADVANCED_FACE('',(#1339),#333,.T.);
#12870=ADVANCED_FACE('',(#1340),#334,.F.);
#12871=ADVANCED_FACE('',(#1341),#335,.F.);
#12872=ADVANCED_FACE('',(#1342),#12284,.F.);
#12873=ADVANCED_FACE('',(#1343),#182,.F.);
#12874=ADVANCED_FACE('',(#1344),#12285,.F.);
#12875=ADVANCED_FACE('',(#1345,#413),#559,.F.);
#12876=ADVANCED_FACE('',(#1346,#414),#560,.F.);
#12877=ADVANCED_FACE('',(#1347),#56,.T.);
#12878=ADVANCED_FACE('',(#1348),#57,.T.);
#12879=ADVANCED_FACE('',(#1349),#58,.T.);
#12880=ADVANCED_FACE('',(#1350),#59,.T.);
#12881=ADVANCED_FACE('',(#1351),#60,.T.);
#12882=ADVANCED_FACE('',(#1352),#61,.T.);
#12883=ADVANCED_FACE('',(#1353),#62,.T.);
#12884=ADVANCED_FACE('',(#1354),#63,.T.);
#12885=ADVANCED_FACE('',(#1355),#12286,.F.);
#12886=ADVANCED_FACE('',(#1356),#183,.T.);
#12887=ADVANCED_FACE('',(#1357),#12287,.T.);
#12888=ADVANCED_FACE('',(#1358),#184,.T.);
#12889=ADVANCED_FACE('',(#1359),#336,.T.);
#12890=ADVANCED_FACE('',(#1360),#12288,.T.);
#12891=ADVANCED_FACE('',(#1361,#415),#561,.F.);
#12999=CLOSED_SHELL('',(#12840,#12841,#12842,#12843,#12844,#12845,#12846,
#12847,#12848,#12849,#12850,#12851));
#13000=CLOSED_SHELL('',(#12852));
#13001=CLOSED_SHELL('',(#12853,#12854,#12855,#12856,#12857,#12858));
#13002=CLOSED_SHELL('',(#12859,#12860,#12861,#12862,#12863,#12864));
#13003=CLOSED_SHELL('',(#12865,#12866,#12867,#12868,#12869,#12870,#12871,
#12872,#12873,#12874,#12875,#12876));
#13004=CLOSED_SHELL('',(#12877));
#13005=CLOSED_SHELL('',(#12878));
#13006=CLOSED_SHELL('',(#12879));
#13007=CLOSED_SHELL('',(#12880));
#13008=CLOSED_SHELL('',(#12881));
#13009=CLOSED_SHELL('',(#12882));
#13010=CLOSED_SHELL('',(#12883));
#13011=CLOSED_SHELL('',(#12884));
#13012=CLOSED_SHELL('',(#12885,#12886,#12887,#12888,#12889,#12890,#12891));
#13993=AXIS2_PLACEMENT_3D('',#87502,#16530,#16531);
#13994=AXIS2_PLACEMENT_3D('',#87503,#16532,#16533);
#13995=AXIS2_PLACEMENT_3D('',#87505,#16534,#16535);
#13996=AXIS2_PLACEMENT_3D('',#87507,#16536,#16537);
#13997=AXIS2_PLACEMENT_3D('',#87508,#16538,#16539);
#13998=AXIS2_PLACEMENT_3D('',#87509,#16540,#16541);
#13999=AXIS2_PLACEMENT_3D('',#87512,#16542,#16543);
#14000=AXIS2_PLACEMENT_3D('',#87516,#16545,#16546);
#14001=AXIS2_PLACEMENT_3D('',#87517,#16547,#16548);
#14002=AXIS2_PLACEMENT_3D('',#87518,#16549,#16550);
#14003=AXIS2_PLACEMENT_3D('',#87519,#16551,#16552);
#14004=AXIS2_PLACEMENT_3D('',#87522,#16554,#16555);
#14005=AXIS2_PLACEMENT_3D('',#87523,#16556,#16557);
#14006=AXIS2_PLACEMENT_3D('',#87526,#16559,#16560);
#14007=AXIS2_PLACEMENT_3D('',#87527,#16561,#16562);
#14008=AXIS2_PLACEMENT_3D('',#87529,#16563,#16564);
#14009=AXIS2_PLACEMENT_3D('',#87530,#16565,#16566);
#14010=AXIS2_PLACEMENT_3D('',#87531,#16567,#16568);
#14011=AXIS2_PLACEMENT_3D('',#87533,#16569,#16570);
#14012=AXIS2_PLACEMENT_3D('',#87535,#16571,#16572);
#14013=AXIS2_PLACEMENT_3D('',#87536,#16573,#16574);
#14014=AXIS2_PLACEMENT_3D('',#87537,#16575,#16576);
#14015=AXIS2_PLACEMENT_3D('',#87539,#16578,#16579);
#14016=AXIS2_PLACEMENT_3D('',#87542,#16581,#16582);
#14017=AXIS2_PLACEMENT_3D('',#87543,#16583,#16584);
#14018=AXIS2_PLACEMENT_3D('',#87545,#16585,#16586);
#14019=AXIS2_PLACEMENT_3D('',#87546,#16587,#16588);
#14020=AXIS2_PLACEMENT_3D('',#87547,#16589,#16590);
#14021=AXIS2_PLACEMENT_3D('',#87549,#16591,#16592);
#14022=AXIS2_PLACEMENT_3D('',#87550,#16593,#16594);
#14023=AXIS2_PLACEMENT_3D('',#87551,#16595,#16596);
#14024=AXIS2_PLACEMENT_3D('',#87552,#16597,#16598);
#14025=AXIS2_PLACEMENT_3D('',#87553,#16599,#16600);
#14026=AXIS2_PLACEMENT_3D('',#87556,#16601,#16602);
#14027=AXIS2_PLACEMENT_3D('',#87557,#16603,#16604);
#14028=AXIS2_PLACEMENT_3D('',#87559,#16605,#16606);
#14029=AXIS2_PLACEMENT_3D('',#87562,#16608,#16609);
#14030=AXIS2_PLACEMENT_3D('',#87563,#16610,#16611);
#14031=AXIS2_PLACEMENT_3D('',#87565,#16612,#16613);
#14032=AXIS2_PLACEMENT_3D('',#87566,#16614,#16615);
#14033=AXIS2_PLACEMENT_3D('',#87567,#16616,#16617);
#14034=AXIS2_PLACEMENT_3D('',#87570,#16618,#16619);
#14035=AXIS2_PLACEMENT_3D('',#87573,#16621,#16622);
#14036=AXIS2_PLACEMENT_3D('',#87574,#16623,#16624);
#14037=AXIS2_PLACEMENT_3D('',#87575,#16625,#16626);
#14038=AXIS2_PLACEMENT_3D('',#87578,#16628,#16629);
#14039=AXIS2_PLACEMENT_3D('',#87579,#16630,#16631);
#14040=AXIS2_PLACEMENT_3D('',#87580,#16632,#16633);
#14041=AXIS2_PLACEMENT_3D('',#87581,#16634,#16635);
#14042=AXIS2_PLACEMENT_3D('',#87583,#16636,#16637);
#14043=AXIS2_PLACEMENT_3D('',#87586,#16639,#16640);
#14044=AXIS2_PLACEMENT_3D('',#87587,#16641,#16642);
#14045=AXIS2_PLACEMENT_3D('',#87589,#16643,#16644);
#14046=AXIS2_PLACEMENT_3D('',#87592,#16646,#16647);
#14047=AXIS2_PLACEMENT_3D('',#87593,#16648,#16649);
#14048=AXIS2_PLACEMENT_3D('',#87595,#16650,#16651);
#14049=AXIS2_PLACEMENT_3D('',#87596,#16652,#16653);
#14050=AXIS2_PLACEMENT_3D('',#87597,#16654,#16655);
#14051=AXIS2_PLACEMENT_3D('',#87600,#16657,#16658);
#14052=AXIS2_PLACEMENT_3D('',#87601,#16659,#16660);
#14053=AXIS2_PLACEMENT_3D('',#87602,#16661,#16662);
#14054=AXIS2_PLACEMENT_3D('',#87603,#16663,#16664);
#14055=AXIS2_PLACEMENT_3D('',#87605,#16665,#16666);
#14056=AXIS2_PLACEMENT_3D('',#87608,#16668,#16669);
#14057=AXIS2_PLACEMENT_3D('',#87609,#16670,#16671);
#14058=AXIS2_PLACEMENT_3D('',#87612,#16673,#16674);
#14059=AXIS2_PLACEMENT_3D('',#87613,#16675,#16676);
#14060=AXIS2_PLACEMENT_3D('',#87616,#16677,#16678);
#14061=AXIS2_PLACEMENT_3D('',#87619,#16680,#16681);
#14062=AXIS2_PLACEMENT_3D('',#87620,#16682,#16683);
#14063=AXIS2_PLACEMENT_3D('',#87621,#16684,#16685);
#14064=AXIS2_PLACEMENT_3D('',#87624,#16687,#16688);
#14065=AXIS2_PLACEMENT_3D('',#87625,#16689,#16690);
#14066=AXIS2_PLACEMENT_3D('',#87628,#16692,#16693);
#14067=AXIS2_PLACEMENT_3D('',#87629,#16694,#16695);
#14068=AXIS2_PLACEMENT_3D('',#87631,#16696,#16697);
#14069=AXIS2_PLACEMENT_3D('',#87634,#16699,#16700);
#14070=AXIS2_PLACEMENT_3D('',#87635,#16701,#16702);
#14071=AXIS2_PLACEMENT_3D('',#87638,#16703,#16704);
#14072=AXIS2_PLACEMENT_3D('',#87640,#16706,#16707);
#14073=AXIS2_PLACEMENT_3D('',#87641,#16708,#16709);
#14074=AXIS2_PLACEMENT_3D('',#87644,#16711,#16712);
#14075=AXIS2_PLACEMENT_3D('',#87645,#16713,#16714);
#14076=AXIS2_PLACEMENT_3D('',#87647,#16715,#16716);
#14077=AXIS2_PLACEMENT_3D('',#87648,#16717,#16718);
#14078=AXIS2_PLACEMENT_3D('',#87649,#16719,#16720);
#14079=AXIS2_PLACEMENT_3D('',#87651,#16722,#16723);
#14080=AXIS2_PLACEMENT_3D('',#87652,#16724,#16725);
#14081=AXIS2_PLACEMENT_3D('',#87653,#16726,#16727);
#14082=AXIS2_PLACEMENT_3D('',#87656,#16728,#16729);
#14083=AXIS2_PLACEMENT_3D('',#87657,#16730,#16731);
#14084=AXIS2_PLACEMENT_3D('',#87660,#16732,#16733);
#14085=AXIS2_PLACEMENT_3D('',#87661,#16734,#16735);
#14086=AXIS2_PLACEMENT_3D('',#87664,#16736,#16737);
#14087=AXIS2_PLACEMENT_3D('',#87665,#16738,#16739);
#14088=AXIS2_PLACEMENT_3D('',#87668,#16740,#16741);
#14089=AXIS2_PLACEMENT_3D('',#87669,#16742,#16743);
#14090=AXIS2_PLACEMENT_3D('',#87672,#16744,#16745);
#14091=AXIS2_PLACEMENT_3D('',#87673,#16746,#16747);
#14092=AXIS2_PLACEMENT_3D('',#87676,#16748,#16749);
#14093=AXIS2_PLACEMENT_3D('',#87677,#16750,#16751);
#14094=AXIS2_PLACEMENT_3D('',#87680,#16752,#16753);
#14095=AXIS2_PLACEMENT_3D('',#87681,#16754,#16755);
#14096=AXIS2_PLACEMENT_3D('',#87684,#16756,#16757);
#14097=AXIS2_PLACEMENT_3D('',#87685,#16758,#16759);
#14098=AXIS2_PLACEMENT_3D('',#87687,#16760,#16761);
#14099=AXIS2_PLACEMENT_3D('',#87690,#16763,#16764);
#14100=AXIS2_PLACEMENT_3D('',#87691,#16765,#16766);
#14101=AXIS2_PLACEMENT_3D('',#87693,#16767,#16768);
#14102=AXIS2_PLACEMENT_3D('',#87694,#16769,#16770);
#14103=AXIS2_PLACEMENT_3D('',#87695,#16771,#16772);
#14104=AXIS2_PLACEMENT_3D('',#87698,#16774,#16775);
#14105=AXIS2_PLACEMENT_3D('',#87699,#16776,#16777);
#14106=AXIS2_PLACEMENT_3D('',#87701,#16778,#16779);
#14107=AXIS2_PLACEMENT_3D('',#87703,#16780,#16781);
#14108=AXIS2_PLACEMENT_3D('',#87704,#16782,#16783);
#14109=AXIS2_PLACEMENT_3D('',#87705,#16784,#16785);
#14110=AXIS2_PLACEMENT_3D('',#87708,#16786,#16787);
#14111=AXIS2_PLACEMENT_3D('',#87710,#16789,#16790);
#14112=AXIS2_PLACEMENT_3D('',#87711,#16791,#16792);
#14113=AXIS2_PLACEMENT_3D('',#87714,#16794,#16795);
#14114=AXIS2_PLACEMENT_3D('',#87715,#16796,#16797);
#16530=DIRECTION('axis',(0.,0.,1.));
#16531=DIRECTION('refdir',(1.,0.,0.));
#16532=DIRECTION('center_axis',(0.,-1.83697019872103E-16,1.));
#16533=DIRECTION('ref_axis',(0.,-1.,-1.83697019872103E-16));
#16534=DIRECTION('center_axis',(0.,-1.83697019872103E-16,1.));
#16535=DIRECTION('ref_axis',(0.,-1.,-1.83697019872103E-16));
#16536=DIRECTION('center_axis',(1.,1.22464679914735E-16,2.24963967399279E-32));
#16537=DIRECTION('ref_axis',(-1.22464679914735E-16,1.,1.83697019872103E-16));
#16538=DIRECTION('center_axis',(0.,-1.83697019872103E-16,1.));
#16539=DIRECTION('ref_axis',(0.,-1.,-1.83697019872103E-16));
#16540=DIRECTION('center_axis',(0.,1.83697019872103E-16,-1.));
#16541=DIRECTION('ref_axis',(0.,1.,1.83697019872103E-16));
#16542=DIRECTION('center_axis',(0.,-1.83697019872103E-16,1.));
#16543=DIRECTION('ref_axis',(0.,-1.,-1.83697019872103E-16));
#16544=DIRECTION('',(-3.16961915143177E-17,-0.258819045102521,-0.965925826289068));
#16545=DIRECTION('center_axis',(0.,-1.83697019872103E-16,1.));
#16546=DIRECTION('ref_axis',(0.,-1.,-1.83697019872103E-16));
#16547=DIRECTION('center_axis',(0.,-1.83697019872103E-16,1.));
#16548=DIRECTION('ref_axis',(0.,-1.,-1.83697019872103E-16));
#16549=DIRECTION('center_axis',(0.,-1.83697019872103E-16,1.));
#16550=DIRECTION('ref_axis',(0.,-1.,-1.83697019872103E-16));
#16551=DIRECTION('center_axis',(0.,-1.83697019872103E-16,1.));
#16552=DIRECTION('ref_axis',(0.,-1.,-1.83697019872103E-16));
#16553=DIRECTION('',(0.,-1.83697019872103E-16,1.));
#16554=DIRECTION('center_axis',(0.,-1.83697019872103E-16,1.));
#16555=DIRECTION('ref_axis',(0.,-1.,-1.83697019872103E-16));
#16556=DIRECTION('center_axis',(0.,-1.83697019872103E-16,1.));
#16557=DIRECTION('ref_axis',(0.,-1.,-1.83697019872103E-16));
#16558=DIRECTION('',(-3.16961915143176E-17,0.25881904510252,0.965925826289068));
#16559=DIRECTION('center_axis',(0.,-1.83697019872103E-16,1.));
#16560=DIRECTION('ref_axis',(0.,-1.,-1.83697019872103E-16));
#16561=DIRECTION('center_axis',(0.,-1.83697019872103E-16,1.));
#16562=DIRECTION('ref_axis',(0.,-1.,-1.68690289661508E-16));
#16563=DIRECTION('center_axis',(-1.,-1.22464679914735E-16,-2.24963967399279E-32));
#16564=DIRECTION('ref_axis',(-1.22464679914735E-16,1.,2.10862862076885E-16));
#16565=DIRECTION('center_axis',(0.,-1.83697019872103E-16,1.));
#16566=DIRECTION('ref_axis',(0.,-1.,-1.83697019872103E-16));
#16567=DIRECTION('center_axis',(0.,-1.83697019872103E-16,1.));
#16568=DIRECTION('ref_axis',(0.,-1.,-1.42298278189606E-16));
#16569=DIRECTION('center_axis',(0.,-1.83697019872103E-16,1.));
#16570=DIRECTION('ref_axis',(0.,-1.,-1.83697019872103E-16));
#16571=DIRECTION('center_axis',(-1.,-1.22464679914735E-16,-2.24963967399279E-32));
#16572=DIRECTION('ref_axis',(-1.22464679914735E-16,1.,1.77872847737008E-16));
#16573=DIRECTION('center_axis',(0.,-1.83697019872103E-16,1.));
#16574=DIRECTION('ref_axis',(0.,-1.,-1.83697019872103E-16));
#16575=DIRECTION('center_axis',(0.,-1.83697019872103E-16,1.));
#16576=DIRECTION('ref_axis',(0.,-1.,-1.83697019872103E-16));
#16577=DIRECTION('',(0.,1.83697019872103E-16,-1.));
#16578=DIRECTION('center_axis',(0.,-1.83697019872103E-16,1.));
#16579=DIRECTION('ref_axis',(0.,-1.,-1.83697019872103E-16));
#16580=DIRECTION('',(0.,1.83697019872103E-16,-1.));
#16581=DIRECTION('center_axis',(0.,-1.83697019872103E-16,1.));
#16582=DIRECTION('ref_axis',(0.,-1.,-1.83697019872103E-16));
#16583=DIRECTION('center_axis',(0.,-1.83697019872103E-16,1.));
#16584=DIRECTION('ref_axis',(0.,-1.,-1.42298278189606E-16));
#16585=DIRECTION('center_axis',(-1.,-1.22464679914735E-16,-2.24963967399279E-32));
#16586=DIRECTION('ref_axis',(-1.22464679914735E-16,1.,1.77872847737008E-16));
#16587=DIRECTION('center_axis',(0.,-1.83697019872103E-16,1.));
#16588=DIRECTION('ref_axis',(0.,-1.,-1.83697019872103E-16));
#16589=DIRECTION('center_axis',(0.,-1.83697019872103E-16,1.));
#16590=DIRECTION('ref_axis',(0.,-1.,-1.68690289661508E-16));
#16591=DIRECTION('center_axis',(0.,-1.83697019872103E-16,1.));
#16592=DIRECTION('ref_axis',(0.,-1.,-1.83697019872103E-16));
#16593=DIRECTION('center_axis',(-1.,-1.22464679914735E-16,-2.24963967399279E-32));
#16594=DIRECTION('ref_axis',(-1.22464679914735E-16,1.,2.10862862076885E-16));
#16595=DIRECTION('center_axis',(0.,-1.83697019872103E-16,1.));
#16596=DIRECTION('ref_axis',(0.,-1.,-1.83697019872103E-16));
#16597=DIRECTION('center_axis',(0.,1.83697019872103E-16,-1.));
#16598=DIRECTION('ref_axis',(0.,1.,1.83697019872103E-16));
#16599=DIRECTION('center_axis',(-1.,0.,0.));
#16600=DIRECTION('ref_axis',(0.,1.,0.));
#16601=DIRECTION('center_axis',(0.,1.22464679914735E-16,1.));
#16602=DIRECTION('ref_axis',(0.,-1.,1.22464679914735E-16));
#16603=DIRECTION('center_axis',(0.,-1.83697019872103E-16,1.));
#16604=DIRECTION('ref_axis',(0.,-1.,-1.83697019872103E-16));
#16605=DIRECTION('center_axis',(0.,-1.83697019872103E-16,1.));
#16606=DIRECTION('ref_axis',(0.,-1.,-1.83697019872103E-16));
#16607=DIRECTION('',(0.,-1.83697019872103E-16,1.));
#16608=DIRECTION('center_axis',(0.,-1.83697019872103E-16,1.));
#16609=DIRECTION('ref_axis',(0.,-1.,-1.83697019872103E-16));
#16610=DIRECTION('center_axis',(0.,-1.83697019872103E-16,1.));
#16611=DIRECTION('ref_axis',(0.,-1.,-2.03409989752688E-16));
#16612=DIRECTION('center_axis',(-1.,-1.22464679914735E-16,-2.24963967399279E-32));
#16613=DIRECTION('ref_axis',(-1.22464679914735E-16,1.,1.69508324793907E-16));
#16614=DIRECTION('center_axis',(0.,-1.83697019872103E-16,1.));
#16615=DIRECTION('ref_axis',(0.,-1.,-1.83697019872103E-16));
#16616=DIRECTION('center_axis',(0.,1.83697019872103E-16,-1.));
#16617=DIRECTION('ref_axis',(0.,1.,1.83697019872103E-16));
#16618=DIRECTION('center_axis',(0.,-1.83697019872103E-16,1.));
#16619=DIRECTION('ref_axis',(0.,-1.,-1.83697019872103E-16));
#16620=DIRECTION('',(6.12323399573677E-17,0.5,0.866025403784439));
#16621=DIRECTION('center_axis',(0.,-1.83697019872103E-16,1.));
#16622=DIRECTION('ref_axis',(0.,-1.,-1.83697019872103E-16));
#16623=DIRECTION('center_axis',(0.,-1.83697019872103E-16,1.));
#16624=DIRECTION('ref_axis',(0.,-1.,-1.83697019872103E-16));
#16625=DIRECTION('center_axis',(0.,-1.83697019872103E-16,1.));
#16626=DIRECTION('ref_axis',(0.,-1.,-1.83697019872103E-16));
#16627=DIRECTION('',(0.,1.83697019872103E-16,-1.));
#16628=DIRECTION('center_axis',(0.,-1.83697019872103E-16,1.));
#16629=DIRECTION('ref_axis',(0.,-1.,-1.83697019872103E-16));
#16630=DIRECTION('center_axis',(0.,-1.83697019872103E-16,1.));
#16631=DIRECTION('ref_axis',(0.,-1.,-1.83697019872103E-16));
#16632=DIRECTION('center_axis',(0.,1.83697019872103E-16,-1.));
#16633=DIRECTION('ref_axis',(0.,1.,1.83697019872103E-16));
#16634=DIRECTION('center_axis',(0.,-1.83697019872103E-16,1.));
#16635=DIRECTION('ref_axis',(0.,-1.,-1.83697019872103E-16));
#16636=DIRECTION('center_axis',(0.,-1.83697019872103E-16,1.));
#16637=DIRECTION('ref_axis',(0.,-1.,-1.83697019872103E-16));
#16638=DIRECTION('',(0.,1.83697019872103E-16,-1.));
#16639=DIRECTION('center_axis',(0.,-1.83697019872103E-16,1.));
#16640=DIRECTION('ref_axis',(0.,-1.,-1.83697019872103E-16));
#16641=DIRECTION('center_axis',(0.,-1.83697019872103E-16,1.));
#16642=DIRECTION('ref_axis',(0.,-1.,-1.83697019872103E-16));
#16643=DIRECTION('center_axis',(0.,-1.83697019872103E-16,1.));
#16644=DIRECTION('ref_axis',(0.,-1.,-1.83697019872103E-16));
#16645=DIRECTION('',(0.,-1.83697019872103E-16,1.));
#16646=DIRECTION('center_axis',(0.,-1.83697019872103E-16,1.));
#16647=DIRECTION('ref_axis',(0.,-1.,-1.83697019872103E-16));
#16648=DIRECTION('center_axis',(0.,-1.83697019872103E-16,1.));
#16649=DIRECTION('ref_axis',(0.,-1.,-2.03409989752688E-16));
#16650=DIRECTION('center_axis',(0.,-1.83697019872103E-16,1.));
#16651=DIRECTION('ref_axis',(0.,-1.,-1.83697019872103E-16));
#16652=DIRECTION('center_axis',(-1.,-1.22464679914735E-16,-2.24963967399279E-32));
#16653=DIRECTION('ref_axis',(-1.22464679914735E-16,1.,1.69508324793907E-16));
#16654=DIRECTION('center_axis',(0.,-1.83697019872103E-16,1.));
#16655=DIRECTION('ref_axis',(0.,-1.,-1.83697019872103E-16));
#16656=DIRECTION('',(6.12323399573675E-17,-0.499999999999998,-0.86602540378444));
#16657=DIRECTION('center_axis',(0.,-1.83697019872103E-16,1.));
#16658=DIRECTION('ref_axis',(0.,-1.,-1.83697019872103E-16));
#16659=DIRECTION('center_axis',(0.,-1.83697019872103E-16,1.));
#16660=DIRECTION('ref_axis',(0.,-1.,-1.83697019872103E-16));
#16661=DIRECTION('center_axis',(0.,1.83697019872103E-16,-1.));
#16662=DIRECTION('ref_axis',(0.,1.,1.83697019872103E-16));
#16663=DIRECTION('center_axis',(0.,-1.83697019872103E-16,1.));
#16664=DIRECTION('ref_axis',(0.,-1.,-1.83697019872103E-16));
#16665=DIRECTION('center_axis',(0.,-1.83697019872103E-16,1.));
#16666=DIRECTION('ref_axis',(0.,-1.,-1.83697019872103E-16));
#16667=DIRECTION('',(-4.18853873767693E-17,0.342020143325664,0.93969262078591));
#16668=DIRECTION('center_axis',(0.,-1.83697019872103E-16,1.));
#16669=DIRECTION('ref_axis',(0.,-1.,-1.83697019872103E-16));
#16670=DIRECTION('center_axis',(0.,-1.83697019872103E-16,1.));
#16671=DIRECTION('ref_axis',(0.,-1.,-1.83697019872103E-16));
#16672=DIRECTION('',(-8.65956056235486E-17,0.707106781186541,0.707106781186554));
#16673=DIRECTION('center_axis',(0.,-1.83697019872103E-16,1.));
#16674=DIRECTION('ref_axis',(0.,-1.,-1.83697019872103E-16));
#16675=DIRECTION('center_axis',(0.,1.83697019872103E-16,-1.));
#16676=DIRECTION('ref_axis',(0.,1.,1.83697019872103E-16));
#16677=DIRECTION('center_axis',(0.,-1.83697019872103E-16,1.));
#16678=DIRECTION('ref_axis',(0.,-1.,-1.83697019872103E-16));
#16679=DIRECTION('',(6.12323399573668E-17,0.499999999999993,0.866025403784443));
#16680=DIRECTION('center_axis',(0.,-1.83697019872103E-16,1.));
#16681=DIRECTION('ref_axis',(0.,-1.,-1.83697019872103E-16));
#16682=DIRECTION('center_axis',(0.,-1.83697019872103E-16,1.));
#16683=DIRECTION('ref_axis',(0.,-1.,-1.83697019872103E-16));
#16684=DIRECTION('center_axis',(0.,-1.83697019872103E-16,1.));
#16685=DIRECTION('ref_axis',(0.,-1.,-1.83697019872103E-16));
#16686=DIRECTION('',(0.,1.83697019872103E-16,-1.));
#16687=DIRECTION('center_axis',(0.,-1.83697019872103E-16,1.));
#16688=DIRECTION('ref_axis',(0.,-1.,-1.83697019872103E-16));
#16689=DIRECTION('center_axis',(0.,-1.83697019872103E-16,1.));
#16690=DIRECTION('ref_axis',(0.,-1.,-1.83697019872103E-16));
#16691=DIRECTION('',(6.12323399573667E-17,-0.499999999999992,-0.866025403784443));
#16692=DIRECTION('center_axis',(0.,-1.83697019872103E-16,1.));
#16693=DIRECTION('ref_axis',(0.,-1.,-1.83697019872103E-16));
#16694=DIRECTION('center_axis',(0.,1.83697019872103E-16,-1.));
#16695=DIRECTION('ref_axis',(0.,1.,1.83697019872103E-16));
#16696=DIRECTION('center_axis',(0.,-1.83697019872103E-16,1.));
#16697=DIRECTION('ref_axis',(0.,-1.,-1.83697019872103E-16));
#16698=DIRECTION('',(-8.65956056235486E-17,-0.707106781186542,-0.707106781186554));
#16699=DIRECTION('center_axis',(0.,-1.83697019872103E-16,1.));
#16700=DIRECTION('ref_axis',(0.,-1.,-1.83697019872103E-16));
#16701=DIRECTION('center_axis',(0.,1.83697019872103E-16,-1.));
#16702=DIRECTION('ref_axis',(0.,1.,1.83697019872103E-16));
#16703=DIRECTION('center_axis',(0.,-1.83697019872103E-16,1.));
#16704=DIRECTION('ref_axis',(0.,-1.,-1.83697019872103E-16));
#16705=DIRECTION('',(-4.18853873767694E-17,-0.342020143325664,-0.93969262078591));
#16706=DIRECTION('center_axis',(0.,-1.83697019872103E-16,1.));
#16707=DIRECTION('ref_axis',(0.,-1.,-1.83697019872103E-16));
#16708=DIRECTION('center_axis',(0.,-1.83697019872103E-16,1.));
#16709=DIRECTION('ref_axis',(0.,-1.,-1.83697019872103E-16));
#16710=DIRECTION('',(0.,-1.83697019872103E-16,1.));
#16711=DIRECTION('center_axis',(0.,-1.83697019872103E-16,1.));
#16712=DIRECTION('ref_axis',(0.,-1.,-1.83697019872103E-16));
#16713=DIRECTION('center_axis',(0.,-1.83697019872103E-16,1.));
#16714=DIRECTION('ref_axis',(0.,-1.,-1.83697019872103E-16));
#16715=DIRECTION('center_axis',(1.,1.22464679914735E-16,2.24963967399279E-32));
#16716=DIRECTION('ref_axis',(-1.22464679914735E-16,1.,1.83697019872103E-16));
#16717=DIRECTION('center_axis',(0.,-1.83697019872103E-16,1.));
#16718=DIRECTION('ref_axis',(0.,-1.,-1.83697019872103E-16));
#16719=DIRECTION('center_axis',(0.,-1.83697019872103E-16,1.));
#16720=DIRECTION('ref_axis',(0.,-1.,-1.83697019872103E-16));
#16721=DIRECTION('',(0.,-1.83697019872103E-16,1.));
#16722=DIRECTION('center_axis',(0.,-1.83697019872103E-16,1.));
#16723=DIRECTION('ref_axis',(0.,-1.,-1.83697019872103E-16));
#16724=DIRECTION('center_axis',(0.,1.83697019872103E-16,-1.));
#16725=DIRECTION('ref_axis',(0.,1.,1.83697019872103E-16));
#16726=DIRECTION('center_axis',(-0.766044443118977,0.642787609686541,1.1807816831013E-16));
#16727=DIRECTION('ref_axis',(0.642787609686541,0.766044443118977,-4.29769385815623E-17));
#16728=DIRECTION('center_axis',(1.9679694718355E-16,5.0836448945465E-17,
1.));
#16729=DIRECTION('ref_axis',(-0.642787609686541,-0.766044443118977,1.65441618496298E-16));
#16730=DIRECTION('center_axis',(-0.173648177666927,0.984807753012209,1.80906249375285E-16));
#16731=DIRECTION('ref_axis',(0.984807753012209,0.173648177666927,-1.51798367128467E-16));
#16732=DIRECTION('center_axis',(3.01510415625474E-16,-1.3053259863271E-16,
1.));
#16733=DIRECTION('ref_axis',(-0.984807753012209,-0.173648177666927,2.74263047043202E-16));
#16734=DIRECTION('center_axis',(0.500000000000004,0.866025403784436,1.59086285808736E-16));
#16735=DIRECTION('ref_axis',(0.866025403784436,-0.500000000000004,-2.75545529808155E-16));
#16736=DIRECTION('center_axis',(2.65143809681226E-16,-3.36777869765524E-16,
1.));
#16737=DIRECTION('ref_axis',(-0.866025403784436,0.500000000000004,3.9801020972289E-16));
#16738=DIRECTION('center_axis',(0.939692620785911,0.342020143325663,6.28280810651538E-17));
#16739=DIRECTION('ref_axis',(0.342020143325663,-0.939692620785911,-3.56315753906281E-16));
#16740=DIRECTION('center_axis',(1.04713468441923E-16,-4.71394909929066E-16,
1.));
#16741=DIRECTION('ref_axis',(-0.342020143325663,0.939692620785911,4.78780433821016E-16));
#16742=DIRECTION('center_axis',(0.939692620785906,-0.342020143325676,-6.28280810651561E-17));
#16743=DIRECTION('ref_axis',(-0.342020143325676,-0.939692620785906,-3.5631575390628E-16));
#16744=DIRECTION('center_axis',(-1.04713468441927E-16,-4.71394909929065E-16,
1.));
#16745=DIRECTION('ref_axis',(0.342020143325676,0.939692620785906,4.78780433821015E-16));
#16746=DIRECTION('center_axis',(0.499999999999992,-0.866025403784443,-1.59086285808737E-16));
#16747=DIRECTION('ref_axis',(-0.866025403784443,-0.499999999999992,-2.75545529808153E-16));
#16748=DIRECTION('center_axis',(-2.65143809681228E-16,-3.3677786976552E-16,
1.));
#16749=DIRECTION('ref_axis',(0.866025403784443,0.499999999999992,3.98010209722888E-16));
#16750=DIRECTION('center_axis',(-0.173648177666941,-0.984807753012206,-1.80906249375284E-16));
#16751=DIRECTION('ref_axis',(-0.984807753012206,0.173648177666941,-1.51798367128465E-16));
#16752=DIRECTION('center_axis',(-3.01510415625474E-16,-1.30532598632705E-16,
1.));
#16753=DIRECTION('ref_axis',(0.984807753012206,-0.173648177666941,2.742630470432E-16));
#16754=DIRECTION('center_axis',(-0.766044443118986,-0.64278760968653,-1.18078168310128E-16));
#16755=DIRECTION('ref_axis',(-0.64278760968653,0.766044443118986,-4.29769385815605E-17));
#16756=DIRECTION('center_axis',(-1.96796947183547E-16,5.08364489454677E-17,
1.));
#16757=DIRECTION('ref_axis',(0.64278760968653,-0.766044443118986,1.65441618496296E-16));
#16758=DIRECTION('center_axis',(0.,-1.83697019872103E-16,1.));
#16759=DIRECTION('ref_axis',(0.,-1.,-1.83697019872103E-16));
#16760=DIRECTION('center_axis',(0.,-1.83697019872103E-16,1.));
#16761=DIRECTION('ref_axis',(0.,-1.,-1.83697019872103E-16));
#16762=DIRECTION('',(0.,-1.83697019872103E-16,1.));
#16763=DIRECTION('center_axis',(0.,-1.83697019872103E-16,1.));
#16764=DIRECTION('ref_axis',(0.,-1.,-1.83697019872103E-16));
#16765=DIRECTION('center_axis',(0.,-1.83697019872103E-16,1.));
#16766=DIRECTION('ref_axis',(0.,-1.,-2.0795020232313E-16));
#16767=DIRECTION('center_axis',(-1.,-1.22464679914735E-16,-2.24963967399279E-32));
#16768=DIRECTION('ref_axis',(-1.22464679914735E-16,1.,1.73291835269275E-16));
#16769=DIRECTION('center_axis',(0.,-1.83697019872103E-16,1.));
#16770=DIRECTION('ref_axis',(0.,-1.,-1.83697019872103E-16));
#16771=DIRECTION('center_axis',(0.,-1.83697019872103E-16,1.));
#16772=DIRECTION('ref_axis',(0.,-1.,-1.83697019872103E-16));
#16773=DIRECTION('',(0.,1.83697019872103E-16,-1.));
#16774=DIRECTION('center_axis',(0.,-1.83697019872103E-16,1.));
#16775=DIRECTION('ref_axis',(0.,-1.,-1.83697019872103E-16));
#16776=DIRECTION('center_axis',(0.,-1.83697019872103E-16,1.));
#16777=DIRECTION('ref_axis',(0.,-1.,-2.06474247751558E-16));
#16778=DIRECTION('center_axis',(-1.,-1.22464679914735E-16,-2.24963967399279E-32));
#16779=DIRECTION('ref_axis',(-1.22464679914735E-16,1.,1.72061873126299E-16));
#16780=DIRECTION('center_axis',(0.,-1.83697019872103E-16,1.));
#16781=DIRECTION('ref_axis',(0.,-1.,-1.83697019872103E-16));
#16782=DIRECTION('center_axis',(0.,-1.83697019872103E-16,1.));
#16783=DIRECTION('ref_axis',(0.,-1.,-1.83697019872103E-16));
#16784=DIRECTION('center_axis',(0.,1.83697019872103E-16,-1.));
#16785=DIRECTION('ref_axis',(0.,1.,1.83697019872103E-16));
#16786=DIRECTION('center_axis',(0.,-1.83697019872103E-16,1.));
#16787=DIRECTION('ref_axis',(0.,-1.,-1.83697019872103E-16));
#16788=DIRECTION('',(2.12657684957562E-17,0.173648177666917,0.98480775301221));
#16789=DIRECTION('center_axis',(0.,-1.83697019872103E-16,1.));
#16790=DIRECTION('ref_axis',(0.,-1.,-1.83697019872103E-16));
#16791=DIRECTION('center_axis',(0.,-1.83697019872103E-16,1.));
#16792=DIRECTION('ref_axis',(0.,-1.,-1.83697019872103E-16));
#16793=DIRECTION('',(0.,1.83697019872103E-16,-1.));
#16794=DIRECTION('center_axis',(0.,-1.83697019872103E-16,1.));
#16795=DIRECTION('ref_axis',(0.,-1.,-1.83697019872103E-16));
#16796=DIRECTION('center_axis',(0.,-1.83697019872103E-16,1.));
#16797=DIRECTION('ref_axis',(0.,-1.,-1.83697019872103E-16));
#87502=CARTESIAN_POINT('',(0.,0.,0.));
#87503=CARTESIAN_POINT('Origin',(0.,8.67361737988404E-16,-1.84345908510495E-15));
#87504=CARTESIAN_POINT('',(7.64383710467806E-16,6.24166666666667,1.57709296562448));
#87505=CARTESIAN_POINT('Origin',(0.,2.61383781769835E-16,1.57709296562448));
#87506=CARTESIAN_POINT('',(-7.64383710467806E-16,6.24166666666667,-1.57709296562448));
#87507=CARTESIAN_POINT('Origin',(-9.27159680854475E-16,7.57083333333333,
-4.52719563823237E-16));
#87508=CARTESIAN_POINT('Origin',(0.,8.40798337462783E-16,-1.57709296562448));
#87509=CARTESIAN_POINT('Origin',(0.,8.93829624710071E-16,-1.86578184737232));
#87510=CARTESIAN_POINT('',(5.51091059616309E-16,4.5,-1.86578184737232));
#87511=CARTESIAN_POINT('',(-5.51091059616309E-16,-4.5,-1.86578184737232));
#87512=CARTESIAN_POINT('Origin',(0.,8.93829624710071E-16,-1.86578184737232));
#87513=CARTESIAN_POINT('',(-5.81962364344815E-16,-4.75208333333333,-2.80656965511364));
#87514=CARTESIAN_POINT('',(-5.51091059616309E-16,-4.5,-1.86578184737232));
#87515=CARTESIAN_POINT('',(5.97398016709068E-16,4.75208333333333,-2.80656965511364));
#87516=CARTESIAN_POINT('Origin',(0.,1.06664954132416E-15,-2.80656965511364));
#87517=CARTESIAN_POINT('Origin',(0.,1.06664954132416E-15,-2.80656965511364));
#87518=CARTESIAN_POINT('Origin',(0.,8.93829624710071E-16,-1.86578184737232));
#87519=CARTESIAN_POINT('Origin',(0.,0.,3.));
#87520=CARTESIAN_POINT('',(-5.51091059616309E-16,4.5,1.86578184737232));
#87521=CARTESIAN_POINT('',(-5.51091059616309E-16,4.5,3.));
#87522=CARTESIAN_POINT('Origin',(0.,2.08352494522548E-16,1.86578184737232));
#87523=CARTESIAN_POINT('Origin',(0.,3.55325779084578E-17,2.80656965511364));
#87524=CARTESIAN_POINT('',(-5.81962364344815E-16,4.75208333333333,2.80656965511364));
#87525=CARTESIAN_POINT('',(-5.81962364344815E-16,4.75208333333333,2.80656965511364));
#87526=CARTESIAN_POINT('Origin',(0.,3.55325779084578E-17,2.80656965511364));
#87527=CARTESIAN_POINT('Origin',(0.,0.,2.73902412952163));
#87528=CARTESIAN_POINT('',(-6.12833669073321E-16,5.00416666666667,3.));
#87529=CARTESIAN_POINT('Origin',(-6.12833669073322E-16,5.00416666666667,
2.73902412952163));
#87530=CARTESIAN_POINT('Origin',(0.,-1.49799954810032E-31,3.));
#87531=CARTESIAN_POINT('Origin',(0.,0.,2.73902412952163));
#87532=CARTESIAN_POINT('',(-7.32423384024203E-16,5.98069079618829,3.));
#87533=CARTESIAN_POINT('Origin',(0.,-1.96513426654064E-31,3.));
#87534=CARTESIAN_POINT('',(-7.64383710467806E-16,6.24166666666667,2.73902412952163));
#87535=CARTESIAN_POINT('Origin',(-7.32423384024202E-16,5.98069079618829,
2.73902412952163));
#87536=CARTESIAN_POINT('Origin',(0.,4.79404896654054E-17,2.73902412952163));
#87537=CARTESIAN_POINT('Origin',(0.,0.,3.));
#87538=CARTESIAN_POINT('',(-7.64383710467807E-16,6.24166666666667,3.));
#87539=CARTESIAN_POINT('Origin',(0.,0.,3.));
#87540=CARTESIAN_POINT('',(-7.64383710467806E-16,6.24166666666667,-2.73902412952163));
#87541=CARTESIAN_POINT('',(-7.64383710467807E-16,6.24166666666667,3.));
#87542=CARTESIAN_POINT('Origin',(0.,1.05424162956721E-15,-2.73902412952163));
#87543=CARTESIAN_POINT('Origin',(0.,8.67361737988404E-16,-2.73902412952163));
#87544=CARTESIAN_POINT('',(-7.32423384024202E-16,5.98069079618829,-3.));
#87545=CARTESIAN_POINT('Origin',(-7.32423384024202E-16,5.98069079618829,
-2.73902412952163));
#87546=CARTESIAN_POINT('Origin',(0.,1.10218211923262E-15,-3.));
#87547=CARTESIAN_POINT('Origin',(0.,8.67361737988404E-16,-2.73902412952163));
#87548=CARTESIAN_POINT('',(-6.12833669073321E-16,5.00416666666667,-3.));
#87549=CARTESIAN_POINT('Origin',(0.,1.10218211923262E-15,-3.));
#87550=CARTESIAN_POINT('Origin',(-6.12833669073322E-16,5.00416666666667,
-2.73902412952163));
#87551=CARTESIAN_POINT('Origin',(0.,5.00416666666667,-3.));
#87552=CARTESIAN_POINT('Origin',(0.,5.00416666666667,3.));
#87553=CARTESIAN_POINT('Origin',(0.,7.57083333333333,-5.42416478122349E-16));
#87554=CARTESIAN_POINT('',(-2.0625,7.57083333333333,-5.42416478122349E-16));
#87555=CARTESIAN_POINT('',(2.0625,7.57083333333333,-5.42416478122349E-16));
#87556=CARTESIAN_POINT('Origin',(0.,7.57083333333333,-5.42416478122349E-16));
#87557=CARTESIAN_POINT('Origin',(0.,0.,3.));
#87558=CARTESIAN_POINT('',(-7.91325940049048E-16,6.46166666666667,2.0625));
#87559=CARTESIAN_POINT('Origin',(0.,1.72215956130097E-16,2.0625));
#87560=CARTESIAN_POINT('',(-7.91325940049048E-16,6.46166666666667,2.956));
#87561=CARTESIAN_POINT('',(-7.91325940049049E-16,6.46166666666667,3.));
#87562=CARTESIAN_POINT('Origin',(0.,8.08266887437239E-18,2.956));
#87563=CARTESIAN_POINT('Origin',(0.,0.,2.956));
#87564=CARTESIAN_POINT('',(-7.96714385965296E-16,6.50566666666666,3.));
#87565=CARTESIAN_POINT('Origin',(-7.96714385965296E-16,6.50566666666666,
2.956));
#87566=CARTESIAN_POINT('Origin',(0.,-9.91324452525291E-32,3.));
#87567=CARTESIAN_POINT('Origin',(0.,3.4998982877922E-17,2.80947441116742));
#87568=CARTESIAN_POINT('',(1.08993565124114E-15,8.9,2.80947441116742));
#87569=CARTESIAN_POINT('',(-1.08993565124114E-15,-8.9,2.80947441116742));
#87570=CARTESIAN_POINT('Origin',(0.,3.4998982877922E-17,2.80947441116742));
#87571=CARTESIAN_POINT('',(-1.07646453645052E-15,-8.79,3.));
#87572=CARTESIAN_POINT('',(-1.08993565124114E-15,-8.9,2.80947441116742));
#87573=CARTESIAN_POINT('Origin',(0.,-1.01714425032945E-31,3.));
#87574=CARTESIAN_POINT('Origin',(0.,3.4998982877922E-17,2.80947441116742));
#87575=CARTESIAN_POINT('Origin',(0.,0.,3.));
#87576=CARTESIAN_POINT('',(-1.08993565124114E-15,8.9,2.0625));
#87577=CARTESIAN_POINT('',(-1.08993565124114E-15,8.9,3.));
#87578=CARTESIAN_POINT('Origin',(0.,1.72215956130097E-16,2.0625));
#87579=CARTESIAN_POINT('Origin',(0.,8.9,2.0625));
#87580=CARTESIAN_POINT('Origin',(0.,8.79,3.));
#87581=CARTESIAN_POINT('Origin',(0.,0.,3.));
#87582=CARTESIAN_POINT('',(-1.08993565124114E-15,8.9,-2.0625));
#87583=CARTESIAN_POINT('Origin',(0.,9.29966163102522E-16,-2.0625));
#87584=CARTESIAN_POINT('',(-1.08993565124114E-15,8.9,-2.80947441116743));
#87585=CARTESIAN_POINT('',(-1.08993565124114E-15,8.9,3.));
#87586=CARTESIAN_POINT('Origin',(0.,1.0671831363547E-15,-2.80947441116743));
#87587=CARTESIAN_POINT('Origin',(0.,0.,3.));
#87588=CARTESIAN_POINT('',(-7.91325940049048E-16,6.46166666666667,-2.956));
#87589=CARTESIAN_POINT('Origin',(0.,1.09409945035825E-15,-2.956));
#87590=CARTESIAN_POINT('',(-7.91325940049048E-16,6.46166666666667,-2.0625));
#87591=CARTESIAN_POINT('',(-7.91325940049049E-16,6.46166666666667,3.));
#87592=CARTESIAN_POINT('Origin',(0.,9.29966163102522E-16,-2.0625));
#87593=CARTESIAN_POINT('Origin',(0.,8.67361737988404E-16,-2.956));
#87594=CARTESIAN_POINT('',(-7.96714385965296E-16,6.50566666666667,-3.));
#87595=CARTESIAN_POINT('Origin',(0.,1.10218211923262E-15,-3.00000000000001));
#87596=CARTESIAN_POINT('Origin',(-7.96714385965296E-16,6.50566666666666,
-2.956));
#87597=CARTESIAN_POINT('Origin',(0.,1.10218211923262E-15,-3.00000000000001));
#87598=CARTESIAN_POINT('',(-1.07646453645052E-15,8.79,-3.));
#87599=CARTESIAN_POINT('',(-1.07646453645052E-15,8.79,-3.00000000000001));
#87600=CARTESIAN_POINT('Origin',(0.,1.10218211923262E-15,-3.00000000000001));
#87601=CARTESIAN_POINT('Origin',(0.,8.79,-3.));
#87602=CARTESIAN_POINT('Origin',(0.,8.9,-2.0625));
#87603=CARTESIAN_POINT('Origin',(0.,2.75545529808154E-17,2.85));
#87604=CARTESIAN_POINT('',(-1.08993565124114E-15,8.9,2.52448092746025));
#87605=CARTESIAN_POINT('Origin',(0.,8.73514365178982E-17,2.52448092746025));
#87606=CARTESIAN_POINT('',(-1.1044451750474E-15,9.01847925309041,2.85));
#87607=CARTESIAN_POINT('',(-1.1044451750474E-15,9.01847925309041,2.85));
#87608=CARTESIAN_POINT('Origin',(0.,2.75545529808154E-17,2.85));
#87609=CARTESIAN_POINT('Origin',(0.,-9.27691267013628E-33,3.));
#87610=CARTESIAN_POINT('',(-1.12281487703461E-15,9.16847925309041,3.));
#87611=CARTESIAN_POINT('',(-1.12281487703461E-15,9.16847925309041,3.));
#87612=CARTESIAN_POINT('Origin',(0.,-9.27691267013628E-33,3.));
#87613=CARTESIAN_POINT('Origin',(0.,5.5109105961631E-17,2.7));
#87614=CARTESIAN_POINT('',(1.22464679914735E-15,10.,2.7));
#87615=CARTESIAN_POINT('',(-1.22464679914735E-15,-10.,2.7));
#87616=CARTESIAN_POINT('Origin',(0.,5.5109105961631E-17,2.7));
#87617=CARTESIAN_POINT('',(-1.20343529437285E-15,-9.82679491924311,3.));
#87618=CARTESIAN_POINT('',(-1.22464679914735E-15,-10.,2.7));
#87619=CARTESIAN_POINT('Origin',(0.,1.29376829386856E-32,3.));
#87620=CARTESIAN_POINT('Origin',(0.,5.5109105961631E-17,2.7));
#87621=CARTESIAN_POINT('Origin',(0.,0.,3.));
#87622=CARTESIAN_POINT('',(-1.22464679914735E-15,10.,-2.7));
#87623=CARTESIAN_POINT('',(-1.22464679914735E-15,10.,3.));
#87624=CARTESIAN_POINT('Origin',(0.,1.04707301327099E-15,-2.7));
#87625=CARTESIAN_POINT('Origin',(0.,1.10218211923262E-15,-3.));
#87626=CARTESIAN_POINT('',(-1.20343529437285E-15,9.82679491924311,-3.));
#87627=CARTESIAN_POINT('',(-1.20343529437285E-15,9.82679491924311,-3.));
#87628=CARTESIAN_POINT('Origin',(0.,1.10218211923262E-15,-3.));
#87629=CARTESIAN_POINT('Origin',(0.,1.0746275662518E-15,-2.85));
#87630=CARTESIAN_POINT('',(-1.1044451750474E-15,-9.0184792530904,-2.85000000000001));
#87631=CARTESIAN_POINT('Origin',(0.,1.0746275662518E-15,-2.85));
#87632=CARTESIAN_POINT('',(-1.12281487703461E-15,-9.1684792530904,-3.00000000000001));
#87633=CARTESIAN_POINT('',(-1.1044451750474E-15,-9.0184792530904,-2.85));
#87634=CARTESIAN_POINT('Origin',(0.,1.10218211923262E-15,-3.));
#87635=CARTESIAN_POINT('Origin',(0.,1.01483068271472E-15,-2.52448092746026));
#87636=CARTESIAN_POINT('',(1.08993565124114E-15,8.9,-2.52448092746025));
#87637=CARTESIAN_POINT('',(-1.08993565124114E-15,-8.9,-2.52448092746026));
#87638=CARTESIAN_POINT('Origin',(0.,1.01483068271472E-15,-2.52448092746026));
#87639=CARTESIAN_POINT('',(-1.08993565124114E-15,-8.9,-2.52448092746026));
#87640=CARTESIAN_POINT('Origin',(0.,1.01483068271472E-15,-2.52448092746026));
#87641=CARTESIAN_POINT('Origin',(0.,0.,3.));
#87642=CARTESIAN_POINT('',(-1.08993565124114E-15,8.9,-1.57709296562448));
#87643=CARTESIAN_POINT('',(-1.08993565124114E-15,8.9,3.));
#87644=CARTESIAN_POINT('Origin',(0.,8.40798337462783E-16,-1.57709296562448));
#87645=CARTESIAN_POINT('Origin',(0.,8.67361737988404E-16,-1.84345908510495E-15));
#87646=CARTESIAN_POINT('',(-1.08993565124114E-15,8.9,1.57709296562448));
#87647=CARTESIAN_POINT('Origin',(-9.27159680854475E-16,7.57083333333333,
-4.52719563823237E-16));
#87648=CARTESIAN_POINT('Origin',(0.,2.61383781769836E-16,1.57709296562448));
#87649=CARTESIAN_POINT('Origin',(0.,0.,3.));
#87650=CARTESIAN_POINT('',(-1.08993565124114E-15,8.9,3.));
#87651=CARTESIAN_POINT('Origin',(0.,9.82679491924311,-3.));
#87652=CARTESIAN_POINT('Origin',(0.,9.82679491924311,3.));
#87653=CARTESIAN_POINT('Origin',(4.86643786166852,5.79959480477993,-8.67787717300259E-16));
#87654=CARTESIAN_POINT('',(3.28647119773563,7.12534424975842,-6.24251495160616E-16));
#87655=CARTESIAN_POINT('',(6.44640452560141,4.47384535980144,-1.1113239394399E-15));
#87656=CARTESIAN_POINT('Origin',(4.86643786166852,5.79959480477993,-8.67787717300259E-16));
#87657=CARTESIAN_POINT('Origin',(7.45581536342993,1.31466141175336,-1.69165661592412E-15));
#87658=CARTESIAN_POINT('',(7.09766599699189,3.34582740234104,-1.31853747658759E-15));
#87659=CARTESIAN_POINT('',(7.81396472986797,-0.716504578834321,-2.06477575526065E-15));
#87660=CARTESIAN_POINT('Origin',(7.45581536342993,1.31466141175336,-1.69165661592412E-15));
#87661=CARTESIAN_POINT('Origin',(6.55653399448467,-3.7854166666667,-2.62852576004492E-15));
#87662=CARTESIAN_POINT('',(7.58778399448468,-1.9992392713613,-2.3004102955644E-15));
#87663=CARTESIAN_POINT('',(5.52528399448466,-5.5715940619721,-2.95664122452544E-15));
#87664=CARTESIAN_POINT('Origin',(6.55653399448467,-3.7854166666667,-2.62852576004492E-15));
#87665=CARTESIAN_POINT('Origin',(2.58937750176137,-7.11425621653333,-3.24002366498782E-15));
#87666=CARTESIAN_POINT('',(4.52749353213231,-6.40883967092415,-3.11044074779094E-15));
#87667=CARTESIAN_POINT('',(0.651261471390429,-7.81967276214251,-3.3696065821847E-15));
#87668=CARTESIAN_POINT('Origin',(2.58937750176137,-7.11425621653333,-3.24002366498782E-15));
#87669=CARTESIAN_POINT('Origin',(-2.58937750176147,-7.1142562165333,-3.24002366498781E-15));
#87670=CARTESIAN_POINT('',(-0.651261471390539,-7.81967276214251,-3.36960658218469E-15));
#87671=CARTESIAN_POINT('',(-4.5274935321324,-6.40883967092409,-3.11044074779093E-15));
#87672=CARTESIAN_POINT('Origin',(-2.58937750176147,-7.1142562165333,-3.24002366498781E-15));
#87673=CARTESIAN_POINT('Origin',(-6.55653399448472,-3.78541666666661,-2.62852576004491E-15));
#87674=CARTESIAN_POINT('',(-5.52528399448474,-5.57159406197203,-2.95664122452543E-15));
#87675=CARTESIAN_POINT('',(-7.5877839944847,-1.9992392713612,-2.30041029556439E-15));
#87676=CARTESIAN_POINT('Origin',(-6.55653399448472,-3.78541666666661,-2.62852576004491E-15));
#87677=CARTESIAN_POINT('Origin',(-7.45581536342991,1.31466141175346,-1.6916566159241E-15));
#87678=CARTESIAN_POINT('',(-7.81396472986797,-0.716504578834215,-2.06477575526062E-15));
#87679=CARTESIAN_POINT('',(-7.09766599699184,3.34582740234114,-1.31853747658758E-15));
#87680=CARTESIAN_POINT('Origin',(-7.45581536342991,1.31466141175346,-1.6916566159241E-15));
#87681=CARTESIAN_POINT('Origin',(-4.86643786166844,5.79959480477999,-8.67787717300247E-16));
#87682=CARTESIAN_POINT('',(-6.44640452560135,4.47384535980152,-1.11132393943989E-15));
#87683=CARTESIAN_POINT('',(-3.28647119773553,7.12534424975846,-6.24251495160608E-16));
#87684=CARTESIAN_POINT('Origin',(-4.86643786166844,5.79959480477999,-8.67787717300247E-16));
#87685=CARTESIAN_POINT('Origin',(0.,0.,3.));
#87686=CARTESIAN_POINT('',(-7.64383710467806E-16,6.24166666666667,2.0625));
#87687=CARTESIAN_POINT('Origin',(0.,1.72215956130097E-16,2.0625));
#87688=CARTESIAN_POINT('',(-7.64383710467806E-16,6.24166666666667,2.9175));
#87689=CARTESIAN_POINT('',(-7.64383710467807E-16,6.24166666666667,3.));
#87690=CARTESIAN_POINT('Origin',(0.,1.51550041394482E-17,2.9175));
#87691=CARTESIAN_POINT('Origin',(0.,0.,2.9175));
#87692=CARTESIAN_POINT('',(-7.84590382653737E-16,6.40666666666666,2.9175));
#87693=CARTESIAN_POINT('Origin',(-7.74487046560772E-16,6.32416666666667,
2.9175));
#87694=CARTESIAN_POINT('Origin',(0.,1.51550041394483E-17,2.9175));
#87695=CARTESIAN_POINT('Origin',(0.,0.,3.));
#87696=CARTESIAN_POINT('',(-7.84590382653738E-16,6.40666666666667,2.8925));
#87697=CARTESIAN_POINT('',(-7.84590382653738E-16,6.40666666666667,3.));
#87698=CARTESIAN_POINT('Origin',(0.,1.97474296362508E-17,2.8925));
#87699=CARTESIAN_POINT('Origin',(0.,0.,2.8925));
#87700=CARTESIAN_POINT('',(-7.90156322781782E-16,6.45211601689499,2.8964763029096));
#87701=CARTESIAN_POINT('Origin',(-7.87394654311583E-16,6.42956528249449,
2.8925));
#87702=CARTESIAN_POINT('',(7.90741131415415E-16,-6.45211601689499,2.8964763029096));
#87703=CARTESIAN_POINT('Origin',(0.,1.9016994641649E-17,2.8964763029096));
#87704=CARTESIAN_POINT('Origin',(0.,1.9016994641649E-17,2.8964763029096));
#87705=CARTESIAN_POINT('Origin',(0.,2.89668383572898E-17,2.84231187649393));
#87706=CARTESIAN_POINT('',(7.91325940049048E-16,6.46166666666667,2.84231187649393));
#87707=CARTESIAN_POINT('',(-7.91325940049049E-16,-6.46166666666667,2.84231187649393));
#87708=CARTESIAN_POINT('Origin',(0.,2.89668383572898E-17,2.84231187649393));
#87709=CARTESIAN_POINT('',(-7.91325940049049E-16,-6.46166666666667,2.84231187649393));
#87710=CARTESIAN_POINT('Origin',(0.,2.89668383572898E-17,2.84231187649393));
#87711=CARTESIAN_POINT('Origin',(0.,0.,3.));
#87712=CARTESIAN_POINT('',(-7.91325940049048E-16,6.46166666666667,2.0625));
#87713=CARTESIAN_POINT('',(-7.91325940049049E-16,6.46166666666667,3.));
#87714=CARTESIAN_POINT('Origin',(0.,1.72215956130097E-16,2.0625));
#87715=CARTESIAN_POINT('Origin',(0.,6.24166666666667,2.0625));
#88470=UNCERTAINTY_MEASURE_WITH_UNIT(LENGTH_MEASURE(0.01),#88484,
'DISTANCE_ACCURACY_VALUE',
'Maximum model space distance between geometric entities at asserted c
onnectivities');
#88472=UNCERTAINTY_MEASURE_WITH_UNIT(LENGTH_MEASURE(0.01),#88484,
'DISTANCE_ACCURACY_VALUE',
'Maximum model space distance between geometric entities at asserted c
onnectivities');
#88481=(
GEOMETRIC_REPRESENTATION_CONTEXT(3)
GLOBAL_UNCERTAINTY_ASSIGNED_CONTEXT((#88470))
GLOBAL_UNIT_ASSIGNED_CONTEXT((#88484,#88486,#88487))
REPRESENTATION_CONTEXT('','3D')
);
#88483=(
GEOMETRIC_REPRESENTATION_CONTEXT(3)
GLOBAL_UNCERTAINTY_ASSIGNED_CONTEXT((#88472))
GLOBAL_UNIT_ASSIGNED_CONTEXT((#88484,#88486,#88487))
REPRESENTATION_CONTEXT('','3D')
);
#88484=(
LENGTH_UNIT()
NAMED_UNIT(*)
SI_UNIT(.MILLI.,.METRE.)
);
#88486=(
NAMED_UNIT(*)
PLANE_ANGLE_UNIT()
SI_UNIT($,.RADIAN.)
);
#88487=(
NAMED_UNIT(*)
SI_UNIT($,.STERADIAN.)
SOLID_ANGLE_UNIT()
);
#88496=SHAPE_DEFINITION_REPRESENTATION(#88506,#88527);
#88506=PRODUCT_DEFINITION_SHAPE('',$,#88538);
#88527=SHAPE_REPRESENTATION('',(#13993),#88481);
#88529=PRODUCT_DEFINITION_CONTEXT('part definition',#88561,'design');
#88538=PRODUCT_DEFINITION(
'Permanently Lubricated 440C Stainless Steel Ball Bearing',
'Permanently Lubricated 440C Stainless Steel Ball Bearing',#88548,#88529);
#88548=PRODUCT_DEFINITION_FORMATION('',$,#88571);
#88561=APPLICATION_CONTEXT(
'Core Data for Automotive Mechanical Design Process');
#88562=PRODUCT_CONTEXT('part definition',#88561,'mechanical');
#88571=PRODUCT(
'Permanently Lubricated 440C Stainless Steel Ball Bearing',
'Permanently Lubricated 440C Stainless Steel Ball Bearing',$,(#88562));
#88574=PRESENTATION_STYLE_ASSIGNMENT((#88576));
#88576=SURFACE_STYLE_USAGE(.BOTH.,#88578);
#88578=SURFACE_SIDE_STYLE('',(#88580));
#88580=SURFACE_STYLE_FILL_AREA(#88582);
#88582=FILL_AREA_STYLE('Opaque(160,160,160)',(#88584));
#88584=FILL_AREA_STYLE_COLOUR('Opaque(160,160,160)',#88586);
#88586=COLOUR_RGB('Opaque(160,160,160)', 0.66274510, 0.83137255, 0.94901961);
ENDSEC;
END-ISO-10303-21;
